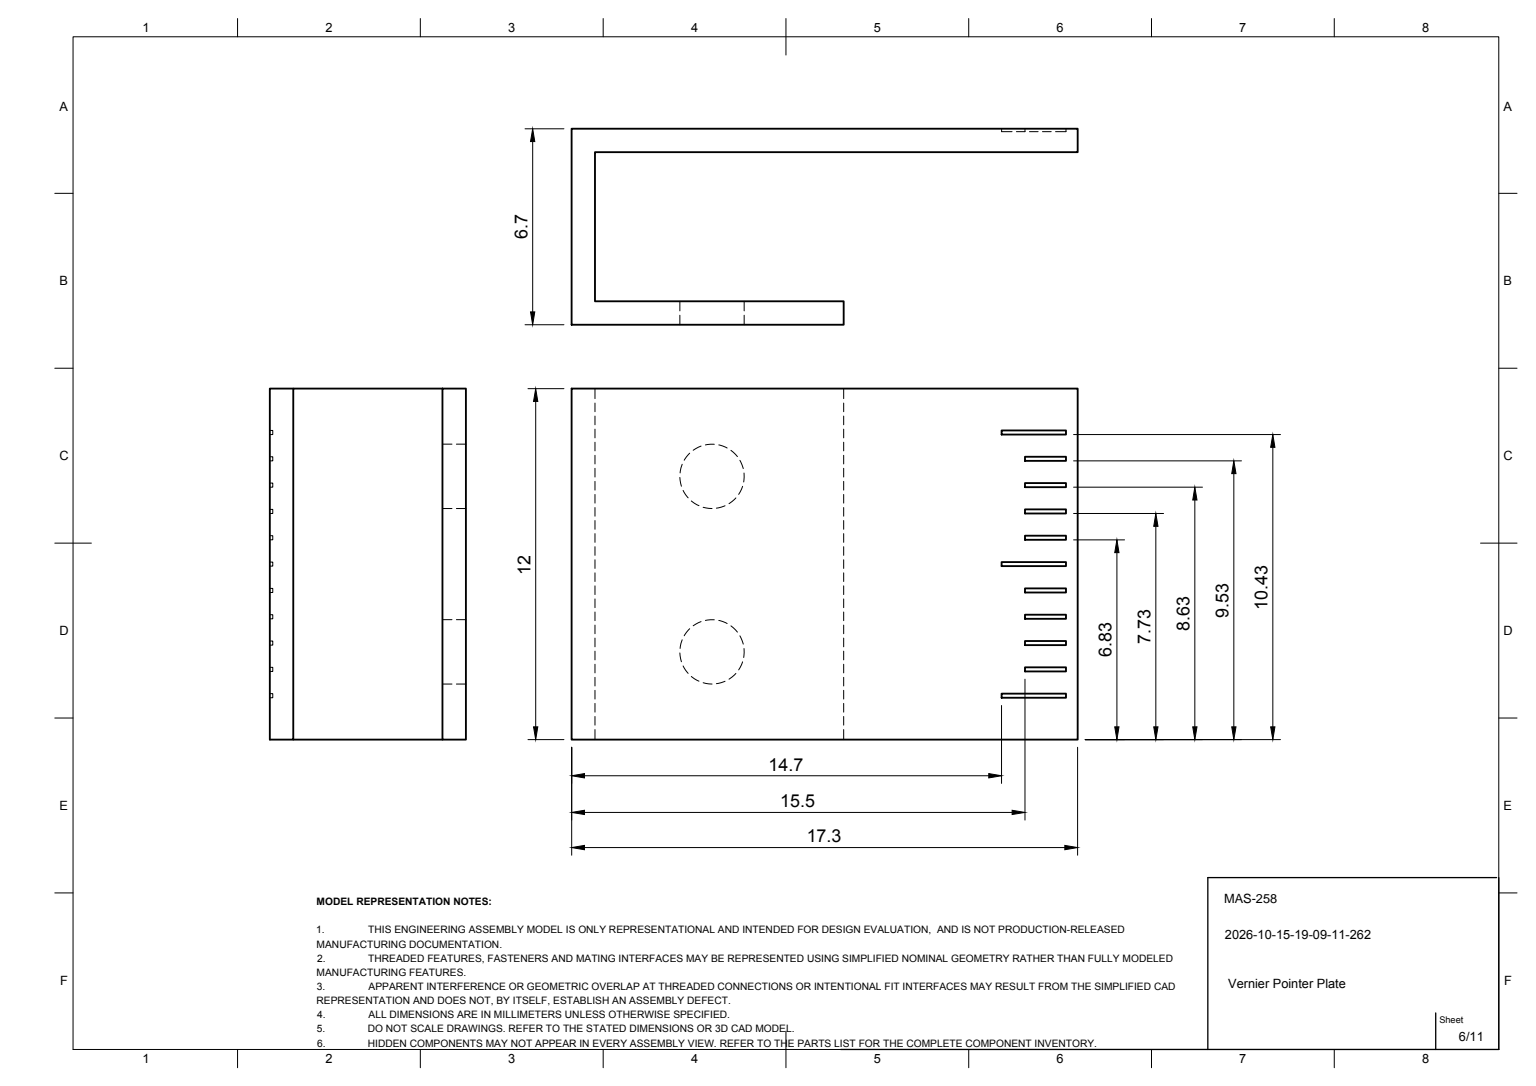
ISO-10303-21;
HEADER;
/* Generated by software containing ST-Developer
 * from STEP Tools, Inc. (www.steptools.com) 
 */

FILE_DESCRIPTION(
/* description */ (''),
/* implementation_level */ '2;1');

FILE_NAME(
/* name */ 'Vernier Pointer Plate.step',
/* time_stamp */ '2026-10-15T12:29:06-07:00',
/* author */ (''),
/* organization */ (''),
/* preprocessor_version */ 'ST-DEVELOPER v20.2',
/* originating_system */ 'Autodesk Translation Framework v15.15.0.0',
/* authorisation */ '');

FILE_SCHEMA (('AUTOMOTIVE_DESIGN { 1 0 10303 214 3 1 1 }'));
ENDSEC;

DATA;
#10=MECHANICAL_DESIGN_GEOMETRIC_PRESENTATION_REPRESENTATION('',(#1745),#135282);
#1719=SHAPE_REPRESENTATION_RELATIONSHIP('SRR','None',#135343,#1732);
#1732=ADVANCED_BREP_SHAPE_REPRESENTATION('',(#1758),#135275);
#1745=STYLED_ITEM('',(#135417),#1758);
#1758=MANIFOLD_SOLID_BREP('Body1',#32081);
#1846=CYLINDRICAL_SURFACE('',#33343,1.1);
#1847=CYLINDRICAL_SURFACE('',#33346,1.1);
#2195=FACE_BOUND('',#6494,.T.);
#2196=FACE_BOUND('',#6495,.T.);
#2197=FACE_BOUND('',#6498,.T.);
#2198=FACE_BOUND('',#6499,.T.);
#2199=FACE_BOUND('',#6504,.T.);
#2200=FACE_BOUND('',#6505,.T.);
#2201=FACE_BOUND('',#6506,.T.);
#2202=FACE_BOUND('',#6507,.T.);
#2203=FACE_BOUND('',#6508,.T.);
#2204=FACE_BOUND('',#6509,.T.);
#2205=FACE_BOUND('',#6510,.T.);
#2206=FACE_BOUND('',#6511,.T.);
#2207=FACE_BOUND('',#6512,.T.);
#2208=FACE_BOUND('',#6513,.T.);
#2209=FACE_BOUND('',#6514,.T.);
#2961=PLANE('',#33288);
#2962=PLANE('',#33289);
#2963=PLANE('',#33290);
#2964=PLANE('',#33291);
#2965=PLANE('',#33292);
#2966=PLANE('',#33293);
#2967=PLANE('',#33294);
#2968=PLANE('',#33295);
#2969=PLANE('',#33296);
#2970=PLANE('',#33297);
#2971=PLANE('',#33298);
#2972=PLANE('',#33299);
#2973=PLANE('',#33300);
#2974=PLANE('',#33301);
#2975=PLANE('',#33302);
#2976=PLANE('',#33303);
#2977=PLANE('',#33304);
#2978=PLANE('',#33305);
#2979=PLANE('',#33306);
#2980=PLANE('',#33307);
#2981=PLANE('',#33308);
#2982=PLANE('',#33309);
#2983=PLANE('',#33310);
#2984=PLANE('',#33311);
#2985=PLANE('',#33312);
#2986=PLANE('',#33313);
#2987=PLANE('',#33314);
#2988=PLANE('',#33315);
#2989=PLANE('',#33316);
#2990=PLANE('',#33317);
#2991=PLANE('',#33318);
#2992=PLANE('',#33319);
#2993=PLANE('',#33320);
#2994=PLANE('',#33321);
#2995=PLANE('',#33322);
#2996=PLANE('',#33323);
#2997=PLANE('',#33324);
#2998=PLANE('',#33325);
#2999=PLANE('',#33326);
#3000=PLANE('',#33327);
#3001=PLANE('',#33328);
#3002=PLANE('',#33329);
#3003=PLANE('',#33330);
#3004=PLANE('',#33331);
#3005=PLANE('',#33332);
#3006=PLANE('',#33333);
#3007=PLANE('',#33334);
#3008=PLANE('',#33335);
#3009=PLANE('',#33336);
#3010=PLANE('',#33337);
#3011=PLANE('',#33338);
#3012=PLANE('',#33339);
#3013=PLANE('',#33340);
#3014=PLANE('',#33341);
#3015=PLANE('',#33342);
#3016=PLANE('',#33349);
#3017=PLANE('',#33350);
#3018=PLANE('',#33351);
#3019=PLANE('',#33352);
#3020=PLANE('',#33353);
#3021=PLANE('',#33354);
#3022=PLANE('',#33355);
#3023=PLANE('',#33356);
#3024=PLANE('',#33357);
#3025=PLANE('',#33358);
#4503=FACE_OUTER_BOUND('',#6436,.T.);
#4504=FACE_OUTER_BOUND('',#6437,.T.);
#4505=FACE_OUTER_BOUND('',#6438,.T.);
#4506=FACE_OUTER_BOUND('',#6439,.T.);
#4507=FACE_OUTER_BOUND('',#6440,.T.);
#4508=FACE_OUTER_BOUND('',#6441,.T.);
#4509=FACE_OUTER_BOUND('',#6442,.T.);
#4510=FACE_OUTER_BOUND('',#6443,.T.);
#4511=FACE_OUTER_BOUND('',#6444,.T.);
#4512=FACE_OUTER_BOUND('',#6445,.T.);
#4513=FACE_OUTER_BOUND('',#6446,.T.);
#4514=FACE_OUTER_BOUND('',#6447,.T.);
#4515=FACE_OUTER_BOUND('',#6448,.T.);
#4516=FACE_OUTER_BOUND('',#6449,.T.);
#4517=FACE_OUTER_BOUND('',#6450,.T.);
#4518=FACE_OUTER_BOUND('',#6451,.T.);
#4519=FACE_OUTER_BOUND('',#6452,.T.);
#4520=FACE_OUTER_BOUND('',#6453,.T.);
#4521=FACE_OUTER_BOUND('',#6454,.T.);
#4522=FACE_OUTER_BOUND('',#6455,.T.);
#4523=FACE_OUTER_BOUND('',#6456,.T.);
#4524=FACE_OUTER_BOUND('',#6457,.T.);
#4525=FACE_OUTER_BOUND('',#6458,.T.);
#4526=FACE_OUTER_BOUND('',#6459,.T.);
#4527=FACE_OUTER_BOUND('',#6460,.T.);
#4528=FACE_OUTER_BOUND('',#6461,.T.);
#4529=FACE_OUTER_BOUND('',#6462,.T.);
#4530=FACE_OUTER_BOUND('',#6463,.T.);
#4531=FACE_OUTER_BOUND('',#6464,.T.);
#4532=FACE_OUTER_BOUND('',#6465,.T.);
#4533=FACE_OUTER_BOUND('',#6466,.T.);
#4534=FACE_OUTER_BOUND('',#6467,.T.);
#4535=FACE_OUTER_BOUND('',#6468,.T.);
#4536=FACE_OUTER_BOUND('',#6469,.T.);
#4537=FACE_OUTER_BOUND('',#6470,.T.);
#4538=FACE_OUTER_BOUND('',#6471,.T.);
#4539=FACE_OUTER_BOUND('',#6472,.T.);
#4540=FACE_OUTER_BOUND('',#6473,.T.);
#4541=FACE_OUTER_BOUND('',#6474,.T.);
#4542=FACE_OUTER_BOUND('',#6475,.T.);
#4543=FACE_OUTER_BOUND('',#6476,.T.);
#4544=FACE_OUTER_BOUND('',#6477,.T.);
#4545=FACE_OUTER_BOUND('',#6478,.T.);
#4546=FACE_OUTER_BOUND('',#6479,.T.);
#4547=FACE_OUTER_BOUND('',#6480,.T.);
#4548=FACE_OUTER_BOUND('',#6481,.T.);
#4549=FACE_OUTER_BOUND('',#6482,.T.);
#4550=FACE_OUTER_BOUND('',#6483,.T.);
#4551=FACE_OUTER_BOUND('',#6484,.T.);
#4552=FACE_OUTER_BOUND('',#6485,.T.);
#4553=FACE_OUTER_BOUND('',#6486,.T.);
#4554=FACE_OUTER_BOUND('',#6487,.T.);
#4555=FACE_OUTER_BOUND('',#6488,.T.);
#4556=FACE_OUTER_BOUND('',#6489,.T.);
#4557=FACE_OUTER_BOUND('',#6490,.T.);
#4558=FACE_OUTER_BOUND('',#6491,.T.);
#4559=FACE_OUTER_BOUND('',#6492,.T.);
#4560=FACE_OUTER_BOUND('',#6493,.T.);
#4561=FACE_OUTER_BOUND('',#6496,.T.);
#4562=FACE_OUTER_BOUND('',#6497,.T.);
#4563=FACE_OUTER_BOUND('',#6500,.T.);
#4564=FACE_OUTER_BOUND('',#6501,.T.);
#4565=FACE_OUTER_BOUND('',#6502,.T.);
#4566=FACE_OUTER_BOUND('',#6503,.T.);
#4567=FACE_OUTER_BOUND('',#6515,.T.);
#4568=FACE_OUTER_BOUND('',#6516,.T.);
#4569=FACE_OUTER_BOUND('',#6517,.T.);
#6436=EDGE_LOOP('',(#26862,#26863,#26864,#26865));
#6437=EDGE_LOOP('',(#26866,#26867,#26868,#26869));
#6438=EDGE_LOOP('',(#26870,#26871,#26872,#26873));
#6439=EDGE_LOOP('',(#26874,#26875,#26876,#26877));
#6440=EDGE_LOOP('',(#26878,#26879,#26880,#26881));
#6441=EDGE_LOOP('',(#26882,#26883,#26884,#26885));
#6442=EDGE_LOOP('',(#26886,#26887,#26888,#26889));
#6443=EDGE_LOOP('',(#26890,#26891,#26892,#26893));
#6444=EDGE_LOOP('',(#26894,#26895,#26896,#26897));
#6445=EDGE_LOOP('',(#26898,#26899,#26900,#26901));
#6446=EDGE_LOOP('',(#26902,#26903,#26904,#26905));
#6447=EDGE_LOOP('',(#26906,#26907,#26908,#26909));
#6448=EDGE_LOOP('',(#26910,#26911,#26912,#26913));
#6449=EDGE_LOOP('',(#26914,#26915,#26916,#26917));
#6450=EDGE_LOOP('',(#26918,#26919,#26920,#26921));
#6451=EDGE_LOOP('',(#26922,#26923,#26924,#26925));
#6452=EDGE_LOOP('',(#26926,#26927,#26928,#26929));
#6453=EDGE_LOOP('',(#26930,#26931,#26932,#26933));
#6454=EDGE_LOOP('',(#26934,#26935,#26936,#26937));
#6455=EDGE_LOOP('',(#26938,#26939,#26940,#26941));
#6456=EDGE_LOOP('',(#26942,#26943,#26944,#26945));
#6457=EDGE_LOOP('',(#26946,#26947,#26948,#26949));
#6458=EDGE_LOOP('',(#26950,#26951,#26952,#26953));
#6459=EDGE_LOOP('',(#26954,#26955,#26956,#26957));
#6460=EDGE_LOOP('',(#26958,#26959,#26960,#26961));
#6461=EDGE_LOOP('',(#26962,#26963,#26964,#26965));
#6462=EDGE_LOOP('',(#26966,#26967,#26968,#26969));
#6463=EDGE_LOOP('',(#26970,#26971,#26972,#26973));
#6464=EDGE_LOOP('',(#26974,#26975,#26976,#26977));
#6465=EDGE_LOOP('',(#26978,#26979,#26980,#26981));
#6466=EDGE_LOOP('',(#26982,#26983,#26984,#26985));
#6467=EDGE_LOOP('',(#26986,#26987,#26988,#26989));
#6468=EDGE_LOOP('',(#26990,#26991,#26992,#26993));
#6469=EDGE_LOOP('',(#26994,#26995,#26996,#26997));
#6470=EDGE_LOOP('',(#26998,#26999,#27000,#27001));
#6471=EDGE_LOOP('',(#27002,#27003,#27004,#27005));
#6472=EDGE_LOOP('',(#27006,#27007,#27008,#27009));
#6473=EDGE_LOOP('',(#27010,#27011,#27012,#27013));
#6474=EDGE_LOOP('',(#27014,#27015,#27016,#27017));
#6475=EDGE_LOOP('',(#27018,#27019,#27020,#27021));
#6476=EDGE_LOOP('',(#27022,#27023,#27024,#27025));
#6477=EDGE_LOOP('',(#27026,#27027,#27028,#27029));
#6478=EDGE_LOOP('',(#27030,#27031,#27032,#27033));
#6479=EDGE_LOOP('',(#27034,#27035,#27036,#27037));
#6480=EDGE_LOOP('',(#27038,#27039,#27040,#27041));
#6481=EDGE_LOOP('',(#27042,#27043,#27044,#27045));
#6482=EDGE_LOOP('',(#27046,#27047,#27048,#27049));
#6483=EDGE_LOOP('',(#27050,#27051,#27052,#27053));
#6484=EDGE_LOOP('',(#27054,#27055,#27056,#27057));
#6485=EDGE_LOOP('',(#27058,#27059,#27060,#27061));
#6486=EDGE_LOOP('',(#27062,#27063,#27064,#27065));
#6487=EDGE_LOOP('',(#27066,#27067,#27068,#27069));
#6488=EDGE_LOOP('',(#27070,#27071,#27072,#27073));
#6489=EDGE_LOOP('',(#27074,#27075,#27076,#27077));
#6490=EDGE_LOOP('',(#27078,#27079,#27080,#27081));
#6491=EDGE_LOOP('',(#27082,#27083,#27084,#27085));
#6492=EDGE_LOOP('',(#27086,#27087,#27088,#27089));
#6493=EDGE_LOOP('',(#27090,#27091,#27092,#27093));
#6494=EDGE_LOOP('',(#27094));
#6495=EDGE_LOOP('',(#27095));
#6496=EDGE_LOOP('',(#27096,#27097,#27098,#27099));
#6497=EDGE_LOOP('',(#27100,#27101,#27102,#27103));
#6498=EDGE_LOOP('',(#27104));
#6499=EDGE_LOOP('',(#27105));
#6500=EDGE_LOOP('',(#27106,#27107,#27108,#27109));
#6501=EDGE_LOOP('',(#27110,#27111,#27112,#27113));
#6502=EDGE_LOOP('',(#27114,#27115,#27116,#27117));
#6503=EDGE_LOOP('',(#27118,#27119,#27120,#27121));
#6504=EDGE_LOOP('',(#27122,#27123,#27124,#27125));
#6505=EDGE_LOOP('',(#27126,#27127,#27128,#27129));
#6506=EDGE_LOOP('',(#27130,#27131,#27132,#27133));
#6507=EDGE_LOOP('',(#27134,#27135,#27136,#27137));
#6508=EDGE_LOOP('',(#27138,#27139,#27140,#27141));
#6509=EDGE_LOOP('',(#27142,#27143,#27144,#27145));
#6510=EDGE_LOOP('',(#27146,#27147,#27148,#27149));
#6511=EDGE_LOOP('',(#27150,#27151,#27152,#27153));
#6512=EDGE_LOOP('',(#27154,#27155,#27156,#27157));
#6513=EDGE_LOOP('',(#27158,#27159,#27160,#27161));
#6514=EDGE_LOOP('',(#27162,#27163,#27164,#27165));
#6515=EDGE_LOOP('',(#27166,#27167,#27168,#27169));
#6516=EDGE_LOOP('',(#27170,#27171,#27172,#27173,#27174,#27175,#27176,#27177));
#6517=EDGE_LOOP('',(#27178,#27179,#27180,#27181,#27182,#27183,#27184,#27185));
#9058=LINE('',#76652,#11895);
#9059=LINE('',#76654,#11896);
#9060=LINE('',#76656,#11897);
#9061=LINE('',#76657,#11898);
#9062=LINE('',#76660,#11899);
#9063=LINE('',#76662,#11900);
#9064=LINE('',#76663,#11901);
#9065=LINE('',#76666,#11902);
#9066=LINE('',#76668,#11903);
#9067=LINE('',#76669,#11904);
#9068=LINE('',#76671,#11905);
#9069=LINE('',#76672,#11906);
#9070=LINE('',#76677,#11907);
#9071=LINE('',#76679,#11908);
#9072=LINE('',#76681,#11909);
#9073=LINE('',#76682,#11910);
#9074=LINE('',#76685,#11911);
#9075=LINE('',#76687,#11912);
#9076=LINE('',#76688,#11913);
#9077=LINE('',#76691,#11914);
#9078=LINE('',#76693,#11915);
#9079=LINE('',#76694,#11916);
#9080=LINE('',#76696,#11917);
#9081=LINE('',#76697,#11918);
#9082=LINE('',#76702,#11919);
#9083=LINE('',#76704,#11920);
#9084=LINE('',#76706,#11921);
#9085=LINE('',#76707,#11922);
#9086=LINE('',#76710,#11923);
#9087=LINE('',#76712,#11924);
#9088=LINE('',#76713,#11925);
#9089=LINE('',#76716,#11926);
#9090=LINE('',#76718,#11927);
#9091=LINE('',#76719,#11928);
#9092=LINE('',#76721,#11929);
#9093=LINE('',#76722,#11930);
#9094=LINE('',#76727,#11931);
#9095=LINE('',#76729,#11932);
#9096=LINE('',#76731,#11933);
#9097=LINE('',#76732,#11934);
#9098=LINE('',#76735,#11935);
#9099=LINE('',#76737,#11936);
#9100=LINE('',#76738,#11937);
#9101=LINE('',#76741,#11938);
#9102=LINE('',#76743,#11939);
#9103=LINE('',#76744,#11940);
#9104=LINE('',#76746,#11941);
#9105=LINE('',#76747,#11942);
#9106=LINE('',#76752,#11943);
#9107=LINE('',#76754,#11944);
#9108=LINE('',#76756,#11945);
#9109=LINE('',#76757,#11946);
#9110=LINE('',#76760,#11947);
#9111=LINE('',#76762,#11948);
#9112=LINE('',#76763,#11949);
#9113=LINE('',#76766,#11950);
#9114=LINE('',#76768,#11951);
#9115=LINE('',#76769,#11952);
#9116=LINE('',#76771,#11953);
#9117=LINE('',#76772,#11954);
#9118=LINE('',#76777,#11955);
#9119=LINE('',#76779,#11956);
#9120=LINE('',#76781,#11957);
#9121=LINE('',#76782,#11958);
#9122=LINE('',#76785,#11959);
#9123=LINE('',#76787,#11960);
#9124=LINE('',#76788,#11961);
#9125=LINE('',#76791,#11962);
#9126=LINE('',#76793,#11963);
#9127=LINE('',#76794,#11964);
#9128=LINE('',#76796,#11965);
#9129=LINE('',#76797,#11966);
#9130=LINE('',#76802,#11967);
#9131=LINE('',#76804,#11968);
#9132=LINE('',#76806,#11969);
#9133=LINE('',#76807,#11970);
#9134=LINE('',#76810,#11971);
#9135=LINE('',#76812,#11972);
#9136=LINE('',#76813,#11973);
#9137=LINE('',#76816,#11974);
#9138=LINE('',#76818,#11975);
#9139=LINE('',#76819,#11976);
#9140=LINE('',#76821,#11977);
#9141=LINE('',#76822,#11978);
#9142=LINE('',#76827,#11979);
#9143=LINE('',#76829,#11980);
#9144=LINE('',#76831,#11981);
#9145=LINE('',#76832,#11982);
#9146=LINE('',#76835,#11983);
#9147=LINE('',#76837,#11984);
#9148=LINE('',#76838,#11985);
#9149=LINE('',#76841,#11986);
#9150=LINE('',#76843,#11987);
#9151=LINE('',#76844,#11988);
#9152=LINE('',#76846,#11989);
#9153=LINE('',#76847,#11990);
#9154=LINE('',#76852,#11991);
#9155=LINE('',#76854,#11992);
#9156=LINE('',#76856,#11993);
#9157=LINE('',#76857,#11994);
#9158=LINE('',#76860,#11995);
#9159=LINE('',#76862,#11996);
#9160=LINE('',#76863,#11997);
#9161=LINE('',#76866,#11998);
#9162=LINE('',#76868,#11999);
#9163=LINE('',#76869,#12000);
#9164=LINE('',#76871,#12001);
#9165=LINE('',#76872,#12002);
#9166=LINE('',#76877,#12003);
#9167=LINE('',#76879,#12004);
#9168=LINE('',#76881,#12005);
#9169=LINE('',#76882,#12006);
#9170=LINE('',#76885,#12007);
#9171=LINE('',#76887,#12008);
#9172=LINE('',#76888,#12009);
#9173=LINE('',#76891,#12010);
#9174=LINE('',#76893,#12011);
#9175=LINE('',#76894,#12012);
#9176=LINE('',#76896,#12013);
#9177=LINE('',#76897,#12014);
#9178=LINE('',#76902,#12015);
#9179=LINE('',#76904,#12016);
#9180=LINE('',#76906,#12017);
#9181=LINE('',#76907,#12018);
#9182=LINE('',#76910,#12019);
#9183=LINE('',#76912,#12020);
#9184=LINE('',#76913,#12021);
#9185=LINE('',#76916,#12022);
#9186=LINE('',#76918,#12023);
#9187=LINE('',#76919,#12024);
#9188=LINE('',#76921,#12025);
#9189=LINE('',#76922,#12026);
#9190=LINE('',#76928,#12027);
#9191=LINE('',#76934,#12028);
#9192=LINE('',#76939,#12029);
#9193=LINE('',#76941,#12030);
#9194=LINE('',#76943,#12031);
#9195=LINE('',#76944,#12032);
#9196=LINE('',#76947,#12033);
#9197=LINE('',#76949,#12034);
#9198=LINE('',#76950,#12035);
#9199=LINE('',#76953,#12036);
#9200=LINE('',#76955,#12037);
#9201=LINE('',#76956,#12038);
#9202=LINE('',#76959,#12039);
#9203=LINE('',#76961,#12040);
#9204=LINE('',#76962,#12041);
#9205=LINE('',#76965,#12042);
#9206=LINE('',#76967,#12043);
#9207=LINE('',#76968,#12044);
#9208=LINE('',#76971,#12045);
#9209=LINE('',#76973,#12046);
#9210=LINE('',#76974,#12047);
#9211=LINE('',#76977,#12048);
#9212=LINE('',#76979,#12049);
#9213=LINE('',#76980,#12050);
#9214=LINE('',#76982,#12051);
#9215=LINE('',#76983,#12052);
#11895=VECTOR('',#38326,10.);
#11896=VECTOR('',#38327,10.);
#11897=VECTOR('',#38328,10.);
#11898=VECTOR('',#38329,10.);
#11899=VECTOR('',#38332,10.);
#11900=VECTOR('',#38333,10.);
#11901=VECTOR('',#38334,10.);
#11902=VECTOR('',#38337,10.);
#11903=VECTOR('',#38338,10.);
#11904=VECTOR('',#38339,10.);
#11905=VECTOR('',#38342,10.);
#11906=VECTOR('',#38343,10.);
#11907=VECTOR('',#38348,10.);
#11908=VECTOR('',#38349,10.);
#11909=VECTOR('',#38350,10.);
#11910=VECTOR('',#38351,10.);
#11911=VECTOR('',#38354,10.);
#11912=VECTOR('',#38355,10.);
#11913=VECTOR('',#38356,10.);
#11914=VECTOR('',#38359,10.);
#11915=VECTOR('',#38360,10.);
#11916=VECTOR('',#38361,10.);
#11917=VECTOR('',#38364,10.);
#11918=VECTOR('',#38365,10.);
#11919=VECTOR('',#38370,10.);
#11920=VECTOR('',#38371,10.);
#11921=VECTOR('',#38372,10.);
#11922=VECTOR('',#38373,10.);
#11923=VECTOR('',#38376,10.);
#11924=VECTOR('',#38377,10.);
#11925=VECTOR('',#38378,10.);
#11926=VECTOR('',#38381,10.);
#11927=VECTOR('',#38382,10.);
#11928=VECTOR('',#38383,10.);
#11929=VECTOR('',#38386,10.);
#11930=VECTOR('',#38387,10.);
#11931=VECTOR('',#38392,10.);
#11932=VECTOR('',#38393,10.);
#11933=VECTOR('',#38394,10.);
#11934=VECTOR('',#38395,10.);
#11935=VECTOR('',#38398,10.);
#11936=VECTOR('',#38399,10.);
#11937=VECTOR('',#38400,10.);
#11938=VECTOR('',#38403,10.);
#11939=VECTOR('',#38404,10.);
#11940=VECTOR('',#38405,10.);
#11941=VECTOR('',#38408,10.);
#11942=VECTOR('',#38409,10.);
#11943=VECTOR('',#38414,10.);
#11944=VECTOR('',#38415,10.);
#11945=VECTOR('',#38416,10.);
#11946=VECTOR('',#38417,10.);
#11947=VECTOR('',#38420,10.);
#11948=VECTOR('',#38421,10.);
#11949=VECTOR('',#38422,10.);
#11950=VECTOR('',#38425,10.);
#11951=VECTOR('',#38426,10.);
#11952=VECTOR('',#38427,10.);
#11953=VECTOR('',#38430,10.);
#11954=VECTOR('',#38431,10.);
#11955=VECTOR('',#38436,10.);
#11956=VECTOR('',#38437,10.);
#11957=VECTOR('',#38438,10.);
#11958=VECTOR('',#38439,10.);
#11959=VECTOR('',#38442,10.);
#11960=VECTOR('',#38443,10.);
#11961=VECTOR('',#38444,10.);
#11962=VECTOR('',#38447,10.);
#11963=VECTOR('',#38448,10.);
#11964=VECTOR('',#38449,10.);
#11965=VECTOR('',#38452,10.);
#11966=VECTOR('',#38453,10.);
#11967=VECTOR('',#38458,10.);
#11968=VECTOR('',#38459,10.);
#11969=VECTOR('',#38460,10.);
#11970=VECTOR('',#38461,10.);
#11971=VECTOR('',#38464,10.);
#11972=VECTOR('',#38465,10.);
#11973=VECTOR('',#38466,10.);
#11974=VECTOR('',#38469,10.);
#11975=VECTOR('',#38470,10.);
#11976=VECTOR('',#38471,10.);
#11977=VECTOR('',#38474,10.);
#11978=VECTOR('',#38475,10.);
#11979=VECTOR('',#38480,10.);
#11980=VECTOR('',#38481,10.);
#11981=VECTOR('',#38482,10.);
#11982=VECTOR('',#38483,10.);
#11983=VECTOR('',#38486,10.);
#11984=VECTOR('',#38487,10.);
#11985=VECTOR('',#38488,10.);
#11986=VECTOR('',#38491,10.);
#11987=VECTOR('',#38492,10.);
#11988=VECTOR('',#38493,10.);
#11989=VECTOR('',#38496,10.);
#11990=VECTOR('',#38497,10.);
#11991=VECTOR('',#38502,10.);
#11992=VECTOR('',#38503,10.);
#11993=VECTOR('',#38504,10.);
#11994=VECTOR('',#38505,10.);
#11995=VECTOR('',#38508,10.);
#11996=VECTOR('',#38509,10.);
#11997=VECTOR('',#38510,10.);
#11998=VECTOR('',#38513,10.);
#11999=VECTOR('',#38514,10.);
#12000=VECTOR('',#38515,10.);
#12001=VECTOR('',#38518,10.);
#12002=VECTOR('',#38519,10.);
#12003=VECTOR('',#38524,10.);
#12004=VECTOR('',#38525,10.);
#12005=VECTOR('',#38526,10.);
#12006=VECTOR('',#38527,10.);
#12007=VECTOR('',#38530,10.);
#12008=VECTOR('',#38531,10.);
#12009=VECTOR('',#38532,10.);
#12010=VECTOR('',#38535,10.);
#12011=VECTOR('',#38536,10.);
#12012=VECTOR('',#38537,10.);
#12013=VECTOR('',#38540,10.);
#12014=VECTOR('',#38541,10.);
#12015=VECTOR('',#38546,10.);
#12016=VECTOR('',#38547,10.);
#12017=VECTOR('',#38548,10.);
#12018=VECTOR('',#38549,10.);
#12019=VECTOR('',#38552,10.);
#12020=VECTOR('',#38553,10.);
#12021=VECTOR('',#38554,10.);
#12022=VECTOR('',#38557,10.);
#12023=VECTOR('',#38558,10.);
#12024=VECTOR('',#38559,10.);
#12025=VECTOR('',#38562,10.);
#12026=VECTOR('',#38563,10.);
#12027=VECTOR('',#38570,1.1);
#12028=VECTOR('',#38577,1.1);
#12029=VECTOR('',#38582,10.);
#12030=VECTOR('',#38583,10.);
#12031=VECTOR('',#38584,10.);
#12032=VECTOR('',#38585,10.);
#12033=VECTOR('',#38588,10.);
#12034=VECTOR('',#38589,10.);
#12035=VECTOR('',#38590,10.);
#12036=VECTOR('',#38593,10.);
#12037=VECTOR('',#38594,10.);
#12038=VECTOR('',#38595,10.);
#12039=VECTOR('',#38598,10.);
#12040=VECTOR('',#38599,10.);
#12041=VECTOR('',#38600,10.);
#12042=VECTOR('',#38603,10.);
#12043=VECTOR('',#38604,10.);
#12044=VECTOR('',#38605,10.);
#12045=VECTOR('',#38608,10.);
#12046=VECTOR('',#38609,10.);
#12047=VECTOR('',#38610,10.);
#12048=VECTOR('',#38613,10.);
#12049=VECTOR('',#38614,10.);
#12050=VECTOR('',#38615,10.);
#12051=VECTOR('',#38618,10.);
#12052=VECTOR('',#38619,10.);
#12928=CIRCLE('',#33344,1.1);
#12929=CIRCLE('',#33345,1.1);
#12930=CIRCLE('',#33347,1.1);
#12931=CIRCLE('',#33348,1.1);
#15209=VERTEX_POINT('',#76650);
#15210=VERTEX_POINT('',#76651);
#15211=VERTEX_POINT('',#76653);
#15212=VERTEX_POINT('',#76655);
#15213=VERTEX_POINT('',#76659);
#15214=VERTEX_POINT('',#76661);
#15215=VERTEX_POINT('',#76665);
#15216=VERTEX_POINT('',#76667);
#15217=VERTEX_POINT('',#76675);
#15218=VERTEX_POINT('',#76676);
#15219=VERTEX_POINT('',#76678);
#15220=VERTEX_POINT('',#76680);
#15221=VERTEX_POINT('',#76684);
#15222=VERTEX_POINT('',#76686);
#15223=VERTEX_POINT('',#76690);
#15224=VERTEX_POINT('',#76692);
#15225=VERTEX_POINT('',#76700);
#15226=VERTEX_POINT('',#76701);
#15227=VERTEX_POINT('',#76703);
#15228=VERTEX_POINT('',#76705);
#15229=VERTEX_POINT('',#76709);
#15230=VERTEX_POINT('',#76711);
#15231=VERTEX_POINT('',#76715);
#15232=VERTEX_POINT('',#76717);
#15233=VERTEX_POINT('',#76725);
#15234=VERTEX_POINT('',#76726);
#15235=VERTEX_POINT('',#76728);
#15236=VERTEX_POINT('',#76730);
#15237=VERTEX_POINT('',#76734);
#15238=VERTEX_POINT('',#76736);
#15239=VERTEX_POINT('',#76740);
#15240=VERTEX_POINT('',#76742);
#15241=VERTEX_POINT('',#76750);
#15242=VERTEX_POINT('',#76751);
#15243=VERTEX_POINT('',#76753);
#15244=VERTEX_POINT('',#76755);
#15245=VERTEX_POINT('',#76759);
#15246=VERTEX_POINT('',#76761);
#15247=VERTEX_POINT('',#76765);
#15248=VERTEX_POINT('',#76767);
#15249=VERTEX_POINT('',#76775);
#15250=VERTEX_POINT('',#76776);
#15251=VERTEX_POINT('',#76778);
#15252=VERTEX_POINT('',#76780);
#15253=VERTEX_POINT('',#76784);
#15254=VERTEX_POINT('',#76786);
#15255=VERTEX_POINT('',#76790);
#15256=VERTEX_POINT('',#76792);
#15257=VERTEX_POINT('',#76800);
#15258=VERTEX_POINT('',#76801);
#15259=VERTEX_POINT('',#76803);
#15260=VERTEX_POINT('',#76805);
#15261=VERTEX_POINT('',#76809);
#15262=VERTEX_POINT('',#76811);
#15263=VERTEX_POINT('',#76815);
#15264=VERTEX_POINT('',#76817);
#15265=VERTEX_POINT('',#76825);
#15266=VERTEX_POINT('',#76826);
#15267=VERTEX_POINT('',#76828);
#15268=VERTEX_POINT('',#76830);
#15269=VERTEX_POINT('',#76834);
#15270=VERTEX_POINT('',#76836);
#15271=VERTEX_POINT('',#76840);
#15272=VERTEX_POINT('',#76842);
#15273=VERTEX_POINT('',#76850);
#15274=VERTEX_POINT('',#76851);
#15275=VERTEX_POINT('',#76853);
#15276=VERTEX_POINT('',#76855);
#15277=VERTEX_POINT('',#76859);
#15278=VERTEX_POINT('',#76861);
#15279=VERTEX_POINT('',#76865);
#15280=VERTEX_POINT('',#76867);
#15281=VERTEX_POINT('',#76875);
#15282=VERTEX_POINT('',#76876);
#15283=VERTEX_POINT('',#76878);
#15284=VERTEX_POINT('',#76880);
#15285=VERTEX_POINT('',#76884);
#15286=VERTEX_POINT('',#76886);
#15287=VERTEX_POINT('',#76890);
#15288=VERTEX_POINT('',#76892);
#15289=VERTEX_POINT('',#76900);
#15290=VERTEX_POINT('',#76901);
#15291=VERTEX_POINT('',#76903);
#15292=VERTEX_POINT('',#76905);
#15293=VERTEX_POINT('',#76909);
#15294=VERTEX_POINT('',#76911);
#15295=VERTEX_POINT('',#76915);
#15296=VERTEX_POINT('',#76917);
#15297=VERTEX_POINT('',#76925);
#15298=VERTEX_POINT('',#76927);
#15299=VERTEX_POINT('',#76931);
#15300=VERTEX_POINT('',#76933);
#15301=VERTEX_POINT('',#76937);
#15302=VERTEX_POINT('',#76938);
#15303=VERTEX_POINT('',#76940);
#15304=VERTEX_POINT('',#76942);
#15305=VERTEX_POINT('',#76946);
#15306=VERTEX_POINT('',#76948);
#15307=VERTEX_POINT('',#76952);
#15308=VERTEX_POINT('',#76954);
#15309=VERTEX_POINT('',#76958);
#15310=VERTEX_POINT('',#76960);
#15311=VERTEX_POINT('',#76964);
#15312=VERTEX_POINT('',#76966);
#15313=VERTEX_POINT('',#76970);
#15314=VERTEX_POINT('',#76972);
#15315=VERTEX_POINT('',#76976);
#15316=VERTEX_POINT('',#76978);
#19282=EDGE_CURVE('',#15209,#15210,#9058,.T.);
#19283=EDGE_CURVE('',#15209,#15211,#9059,.T.);
#19284=EDGE_CURVE('',#15211,#15212,#9060,.T.);
#19285=EDGE_CURVE('',#15210,#15212,#9061,.T.);
#19286=EDGE_CURVE('',#15213,#15209,#9062,.T.);
#19287=EDGE_CURVE('',#15213,#15214,#9063,.T.);
#19288=EDGE_CURVE('',#15214,#15211,#9064,.T.);
#19289=EDGE_CURVE('',#15215,#15213,#9065,.T.);
#19290=EDGE_CURVE('',#15215,#15216,#9066,.T.);
#19291=EDGE_CURVE('',#15216,#15214,#9067,.T.);
#19292=EDGE_CURVE('',#15210,#15215,#9068,.T.);
#19293=EDGE_CURVE('',#15212,#15216,#9069,.T.);
#19294=EDGE_CURVE('',#15217,#15218,#9070,.T.);
#19295=EDGE_CURVE('',#15217,#15219,#9071,.T.);
#19296=EDGE_CURVE('',#15219,#15220,#9072,.T.);
#19297=EDGE_CURVE('',#15218,#15220,#9073,.T.);
#19298=EDGE_CURVE('',#15221,#15217,#9074,.T.);
#19299=EDGE_CURVE('',#15221,#15222,#9075,.T.);
#19300=EDGE_CURVE('',#15222,#15219,#9076,.T.);
#19301=EDGE_CURVE('',#15223,#15221,#9077,.T.);
#19302=EDGE_CURVE('',#15223,#15224,#9078,.T.);
#19303=EDGE_CURVE('',#15224,#15222,#9079,.T.);
#19304=EDGE_CURVE('',#15218,#15223,#9080,.T.);
#19305=EDGE_CURVE('',#15220,#15224,#9081,.T.);
#19306=EDGE_CURVE('',#15225,#15226,#9082,.T.);
#19307=EDGE_CURVE('',#15225,#15227,#9083,.T.);
#19308=EDGE_CURVE('',#15227,#15228,#9084,.T.);
#19309=EDGE_CURVE('',#15226,#15228,#9085,.T.);
#19310=EDGE_CURVE('',#15229,#15225,#9086,.T.);
#19311=EDGE_CURVE('',#15229,#15230,#9087,.T.);
#19312=EDGE_CURVE('',#15230,#15227,#9088,.T.);
#19313=EDGE_CURVE('',#15231,#15229,#9089,.T.);
#19314=EDGE_CURVE('',#15231,#15232,#9090,.T.);
#19315=EDGE_CURVE('',#15232,#15230,#9091,.T.);
#19316=EDGE_CURVE('',#15226,#15231,#9092,.T.);
#19317=EDGE_CURVE('',#15228,#15232,#9093,.T.);
#19318=EDGE_CURVE('',#15233,#15234,#9094,.T.);
#19319=EDGE_CURVE('',#15233,#15235,#9095,.T.);
#19320=EDGE_CURVE('',#15235,#15236,#9096,.T.);
#19321=EDGE_CURVE('',#15234,#15236,#9097,.T.);
#19322=EDGE_CURVE('',#15237,#15233,#9098,.T.);
#19323=EDGE_CURVE('',#15237,#15238,#9099,.T.);
#19324=EDGE_CURVE('',#15238,#15235,#9100,.T.);
#19325=EDGE_CURVE('',#15239,#15237,#9101,.T.);
#19326=EDGE_CURVE('',#15239,#15240,#9102,.T.);
#19327=EDGE_CURVE('',#15240,#15238,#9103,.T.);
#19328=EDGE_CURVE('',#15234,#15239,#9104,.T.);
#19329=EDGE_CURVE('',#15236,#15240,#9105,.T.);
#19330=EDGE_CURVE('',#15241,#15242,#9106,.T.);
#19331=EDGE_CURVE('',#15241,#15243,#9107,.T.);
#19332=EDGE_CURVE('',#15243,#15244,#9108,.T.);
#19333=EDGE_CURVE('',#15242,#15244,#9109,.T.);
#19334=EDGE_CURVE('',#15245,#15241,#9110,.T.);
#19335=EDGE_CURVE('',#15245,#15246,#9111,.T.);
#19336=EDGE_CURVE('',#15246,#15243,#9112,.T.);
#19337=EDGE_CURVE('',#15247,#15245,#9113,.T.);
#19338=EDGE_CURVE('',#15247,#15248,#9114,.T.);
#19339=EDGE_CURVE('',#15248,#15246,#9115,.T.);
#19340=EDGE_CURVE('',#15242,#15247,#9116,.T.);
#19341=EDGE_CURVE('',#15244,#15248,#9117,.T.);
#19342=EDGE_CURVE('',#15249,#15250,#9118,.T.);
#19343=EDGE_CURVE('',#15249,#15251,#9119,.T.);
#19344=EDGE_CURVE('',#15251,#15252,#9120,.T.);
#19345=EDGE_CURVE('',#15250,#15252,#9121,.T.);
#19346=EDGE_CURVE('',#15253,#15249,#9122,.T.);
#19347=EDGE_CURVE('',#15253,#15254,#9123,.T.);
#19348=EDGE_CURVE('',#15254,#15251,#9124,.T.);
#19349=EDGE_CURVE('',#15255,#15253,#9125,.T.);
#19350=EDGE_CURVE('',#15255,#15256,#9126,.T.);
#19351=EDGE_CURVE('',#15256,#15254,#9127,.T.);
#19352=EDGE_CURVE('',#15250,#15255,#9128,.T.);
#19353=EDGE_CURVE('',#15252,#15256,#9129,.T.);
#19354=EDGE_CURVE('',#15257,#15258,#9130,.T.);
#19355=EDGE_CURVE('',#15257,#15259,#9131,.T.);
#19356=EDGE_CURVE('',#15259,#15260,#9132,.T.);
#19357=EDGE_CURVE('',#15258,#15260,#9133,.T.);
#19358=EDGE_CURVE('',#15261,#15257,#9134,.T.);
#19359=EDGE_CURVE('',#15261,#15262,#9135,.T.);
#19360=EDGE_CURVE('',#15262,#15259,#9136,.T.);
#19361=EDGE_CURVE('',#15263,#15261,#9137,.T.);
#19362=EDGE_CURVE('',#15263,#15264,#9138,.T.);
#19363=EDGE_CURVE('',#15264,#15262,#9139,.T.);
#19364=EDGE_CURVE('',#15258,#15263,#9140,.T.);
#19365=EDGE_CURVE('',#15260,#15264,#9141,.T.);
#19366=EDGE_CURVE('',#15265,#15266,#9142,.T.);
#19367=EDGE_CURVE('',#15265,#15267,#9143,.T.);
#19368=EDGE_CURVE('',#15267,#15268,#9144,.T.);
#19369=EDGE_CURVE('',#15266,#15268,#9145,.T.);
#19370=EDGE_CURVE('',#15269,#15265,#9146,.T.);
#19371=EDGE_CURVE('',#15269,#15270,#9147,.T.);
#19372=EDGE_CURVE('',#15270,#15267,#9148,.T.);
#19373=EDGE_CURVE('',#15271,#15269,#9149,.T.);
#19374=EDGE_CURVE('',#15271,#15272,#9150,.T.);
#19375=EDGE_CURVE('',#15272,#15270,#9151,.T.);
#19376=EDGE_CURVE('',#15266,#15271,#9152,.T.);
#19377=EDGE_CURVE('',#15268,#15272,#9153,.T.);
#19378=EDGE_CURVE('',#15273,#15274,#9154,.T.);
#19379=EDGE_CURVE('',#15273,#15275,#9155,.T.);
#19380=EDGE_CURVE('',#15275,#15276,#9156,.T.);
#19381=EDGE_CURVE('',#15274,#15276,#9157,.T.);
#19382=EDGE_CURVE('',#15277,#15273,#9158,.T.);
#19383=EDGE_CURVE('',#15277,#15278,#9159,.T.);
#19384=EDGE_CURVE('',#15278,#15275,#9160,.T.);
#19385=EDGE_CURVE('',#15279,#15277,#9161,.T.);
#19386=EDGE_CURVE('',#15279,#15280,#9162,.T.);
#19387=EDGE_CURVE('',#15280,#15278,#9163,.T.);
#19388=EDGE_CURVE('',#15274,#15279,#9164,.T.);
#19389=EDGE_CURVE('',#15276,#15280,#9165,.T.);
#19390=EDGE_CURVE('',#15281,#15282,#9166,.T.);
#19391=EDGE_CURVE('',#15281,#15283,#9167,.T.);
#19392=EDGE_CURVE('',#15283,#15284,#9168,.T.);
#19393=EDGE_CURVE('',#15282,#15284,#9169,.T.);
#19394=EDGE_CURVE('',#15285,#15281,#9170,.T.);
#19395=EDGE_CURVE('',#15285,#15286,#9171,.T.);
#19396=EDGE_CURVE('',#15286,#15283,#9172,.T.);
#19397=EDGE_CURVE('',#15287,#15285,#9173,.T.);
#19398=EDGE_CURVE('',#15287,#15288,#9174,.T.);
#19399=EDGE_CURVE('',#15288,#15286,#9175,.T.);
#19400=EDGE_CURVE('',#15282,#15287,#9176,.T.);
#19401=EDGE_CURVE('',#15284,#15288,#9177,.T.);
#19402=EDGE_CURVE('',#15289,#15290,#9178,.T.);
#19403=EDGE_CURVE('',#15289,#15291,#9179,.T.);
#19404=EDGE_CURVE('',#15291,#15292,#9180,.T.);
#19405=EDGE_CURVE('',#15290,#15292,#9181,.T.);
#19406=EDGE_CURVE('',#15293,#15289,#9182,.T.);
#19407=EDGE_CURVE('',#15293,#15294,#9183,.T.);
#19408=EDGE_CURVE('',#15294,#15291,#9184,.T.);
#19409=EDGE_CURVE('',#15295,#15293,#9185,.T.);
#19410=EDGE_CURVE('',#15295,#15296,#9186,.T.);
#19411=EDGE_CURVE('',#15296,#15294,#9187,.T.);
#19412=EDGE_CURVE('',#15290,#15295,#9188,.T.);
#19413=EDGE_CURVE('',#15292,#15296,#9189,.T.);
#19414=EDGE_CURVE('',#15297,#15297,#12928,.T.);
#19415=EDGE_CURVE('',#15297,#15298,#9190,.T.);
#19416=EDGE_CURVE('',#15298,#15298,#12929,.T.);
#19417=EDGE_CURVE('',#15299,#15299,#12930,.T.);
#19418=EDGE_CURVE('',#15299,#15300,#9191,.T.);
#19419=EDGE_CURVE('',#15300,#15300,#12931,.T.);
#19420=EDGE_CURVE('',#15301,#15302,#9192,.T.);
#19421=EDGE_CURVE('',#15301,#15303,#9193,.T.);
#19422=EDGE_CURVE('',#15304,#15303,#9194,.T.);
#19423=EDGE_CURVE('',#15302,#15304,#9195,.T.);
#19424=EDGE_CURVE('',#15302,#15305,#9196,.T.);
#19425=EDGE_CURVE('',#15306,#15304,#9197,.T.);
#19426=EDGE_CURVE('',#15305,#15306,#9198,.T.);
#19427=EDGE_CURVE('',#15305,#15307,#9199,.T.);
#19428=EDGE_CURVE('',#15308,#15306,#9200,.T.);
#19429=EDGE_CURVE('',#15307,#15308,#9201,.T.);
#19430=EDGE_CURVE('',#15307,#15309,#9202,.T.);
#19431=EDGE_CURVE('',#15310,#15308,#9203,.T.);
#19432=EDGE_CURVE('',#15309,#15310,#9204,.T.);
#19433=EDGE_CURVE('',#15309,#15311,#9205,.T.);
#19434=EDGE_CURVE('',#15312,#15310,#9206,.T.);
#19435=EDGE_CURVE('',#15311,#15312,#9207,.T.);
#19436=EDGE_CURVE('',#15311,#15313,#9208,.T.);
#19437=EDGE_CURVE('',#15314,#15312,#9209,.T.);
#19438=EDGE_CURVE('',#15313,#15314,#9210,.T.);
#19439=EDGE_CURVE('',#15313,#15315,#9211,.T.);
#19440=EDGE_CURVE('',#15316,#15314,#9212,.T.);
#19441=EDGE_CURVE('',#15315,#15316,#9213,.T.);
#19442=EDGE_CURVE('',#15315,#15301,#9214,.T.);
#19443=EDGE_CURVE('',#15303,#15316,#9215,.T.);
#26862=ORIENTED_EDGE('',*,*,#19282,.F.);
#26863=ORIENTED_EDGE('',*,*,#19283,.T.);
#26864=ORIENTED_EDGE('',*,*,#19284,.T.);
#26865=ORIENTED_EDGE('',*,*,#19285,.F.);
#26866=ORIENTED_EDGE('',*,*,#19286,.F.);
#26867=ORIENTED_EDGE('',*,*,#19287,.T.);
#26868=ORIENTED_EDGE('',*,*,#19288,.T.);
#26869=ORIENTED_EDGE('',*,*,#19283,.F.);
#26870=ORIENTED_EDGE('',*,*,#19289,.F.);
#26871=ORIENTED_EDGE('',*,*,#19290,.T.);
#26872=ORIENTED_EDGE('',*,*,#19291,.T.);
#26873=ORIENTED_EDGE('',*,*,#19287,.F.);
#26874=ORIENTED_EDGE('',*,*,#19292,.F.);
#26875=ORIENTED_EDGE('',*,*,#19285,.T.);
#26876=ORIENTED_EDGE('',*,*,#19293,.T.);
#26877=ORIENTED_EDGE('',*,*,#19290,.F.);
#26878=ORIENTED_EDGE('',*,*,#19293,.F.);
#26879=ORIENTED_EDGE('',*,*,#19284,.F.);
#26880=ORIENTED_EDGE('',*,*,#19288,.F.);
#26881=ORIENTED_EDGE('',*,*,#19291,.F.);
#26882=ORIENTED_EDGE('',*,*,#19294,.F.);
#26883=ORIENTED_EDGE('',*,*,#19295,.T.);
#26884=ORIENTED_EDGE('',*,*,#19296,.T.);
#26885=ORIENTED_EDGE('',*,*,#19297,.F.);
#26886=ORIENTED_EDGE('',*,*,#19298,.F.);
#26887=ORIENTED_EDGE('',*,*,#19299,.T.);
#26888=ORIENTED_EDGE('',*,*,#19300,.T.);
#26889=ORIENTED_EDGE('',*,*,#19295,.F.);
#26890=ORIENTED_EDGE('',*,*,#19301,.F.);
#26891=ORIENTED_EDGE('',*,*,#19302,.T.);
#26892=ORIENTED_EDGE('',*,*,#19303,.T.);
#26893=ORIENTED_EDGE('',*,*,#19299,.F.);
#26894=ORIENTED_EDGE('',*,*,#19304,.F.);
#26895=ORIENTED_EDGE('',*,*,#19297,.T.);
#26896=ORIENTED_EDGE('',*,*,#19305,.T.);
#26897=ORIENTED_EDGE('',*,*,#19302,.F.);
#26898=ORIENTED_EDGE('',*,*,#19305,.F.);
#26899=ORIENTED_EDGE('',*,*,#19296,.F.);
#26900=ORIENTED_EDGE('',*,*,#19300,.F.);
#26901=ORIENTED_EDGE('',*,*,#19303,.F.);
#26902=ORIENTED_EDGE('',*,*,#19306,.F.);
#26903=ORIENTED_EDGE('',*,*,#19307,.T.);
#26904=ORIENTED_EDGE('',*,*,#19308,.T.);
#26905=ORIENTED_EDGE('',*,*,#19309,.F.);
#26906=ORIENTED_EDGE('',*,*,#19310,.F.);
#26907=ORIENTED_EDGE('',*,*,#19311,.T.);
#26908=ORIENTED_EDGE('',*,*,#19312,.T.);
#26909=ORIENTED_EDGE('',*,*,#19307,.F.);
#26910=ORIENTED_EDGE('',*,*,#19313,.F.);
#26911=ORIENTED_EDGE('',*,*,#19314,.T.);
#26912=ORIENTED_EDGE('',*,*,#19315,.T.);
#26913=ORIENTED_EDGE('',*,*,#19311,.F.);
#26914=ORIENTED_EDGE('',*,*,#19316,.F.);
#26915=ORIENTED_EDGE('',*,*,#19309,.T.);
#26916=ORIENTED_EDGE('',*,*,#19317,.T.);
#26917=ORIENTED_EDGE('',*,*,#19314,.F.);
#26918=ORIENTED_EDGE('',*,*,#19317,.F.);
#26919=ORIENTED_EDGE('',*,*,#19308,.F.);
#26920=ORIENTED_EDGE('',*,*,#19312,.F.);
#26921=ORIENTED_EDGE('',*,*,#19315,.F.);
#26922=ORIENTED_EDGE('',*,*,#19318,.F.);
#26923=ORIENTED_EDGE('',*,*,#19319,.T.);
#26924=ORIENTED_EDGE('',*,*,#19320,.T.);
#26925=ORIENTED_EDGE('',*,*,#19321,.F.);
#26926=ORIENTED_EDGE('',*,*,#19322,.F.);
#26927=ORIENTED_EDGE('',*,*,#19323,.T.);
#26928=ORIENTED_EDGE('',*,*,#19324,.T.);
#26929=ORIENTED_EDGE('',*,*,#19319,.F.);
#26930=ORIENTED_EDGE('',*,*,#19325,.F.);
#26931=ORIENTED_EDGE('',*,*,#19326,.T.);
#26932=ORIENTED_EDGE('',*,*,#19327,.T.);
#26933=ORIENTED_EDGE('',*,*,#19323,.F.);
#26934=ORIENTED_EDGE('',*,*,#19328,.F.);
#26935=ORIENTED_EDGE('',*,*,#19321,.T.);
#26936=ORIENTED_EDGE('',*,*,#19329,.T.);
#26937=ORIENTED_EDGE('',*,*,#19326,.F.);
#26938=ORIENTED_EDGE('',*,*,#19329,.F.);
#26939=ORIENTED_EDGE('',*,*,#19320,.F.);
#26940=ORIENTED_EDGE('',*,*,#19324,.F.);
#26941=ORIENTED_EDGE('',*,*,#19327,.F.);
#26942=ORIENTED_EDGE('',*,*,#19330,.F.);
#26943=ORIENTED_EDGE('',*,*,#19331,.T.);
#26944=ORIENTED_EDGE('',*,*,#19332,.T.);
#26945=ORIENTED_EDGE('',*,*,#19333,.F.);
#26946=ORIENTED_EDGE('',*,*,#19334,.F.);
#26947=ORIENTED_EDGE('',*,*,#19335,.T.);
#26948=ORIENTED_EDGE('',*,*,#19336,.T.);
#26949=ORIENTED_EDGE('',*,*,#19331,.F.);
#26950=ORIENTED_EDGE('',*,*,#19337,.F.);
#26951=ORIENTED_EDGE('',*,*,#19338,.T.);
#26952=ORIENTED_EDGE('',*,*,#19339,.T.);
#26953=ORIENTED_EDGE('',*,*,#19335,.F.);
#26954=ORIENTED_EDGE('',*,*,#19340,.F.);
#26955=ORIENTED_EDGE('',*,*,#19333,.T.);
#26956=ORIENTED_EDGE('',*,*,#19341,.T.);
#26957=ORIENTED_EDGE('',*,*,#19338,.F.);
#26958=ORIENTED_EDGE('',*,*,#19341,.F.);
#26959=ORIENTED_EDGE('',*,*,#19332,.F.);
#26960=ORIENTED_EDGE('',*,*,#19336,.F.);
#26961=ORIENTED_EDGE('',*,*,#19339,.F.);
#26962=ORIENTED_EDGE('',*,*,#19342,.F.);
#26963=ORIENTED_EDGE('',*,*,#19343,.T.);
#26964=ORIENTED_EDGE('',*,*,#19344,.T.);
#26965=ORIENTED_EDGE('',*,*,#19345,.F.);
#26966=ORIENTED_EDGE('',*,*,#19346,.F.);
#26967=ORIENTED_EDGE('',*,*,#19347,.T.);
#26968=ORIENTED_EDGE('',*,*,#19348,.T.);
#26969=ORIENTED_EDGE('',*,*,#19343,.F.);
#26970=ORIENTED_EDGE('',*,*,#19349,.F.);
#26971=ORIENTED_EDGE('',*,*,#19350,.T.);
#26972=ORIENTED_EDGE('',*,*,#19351,.T.);
#26973=ORIENTED_EDGE('',*,*,#19347,.F.);
#26974=ORIENTED_EDGE('',*,*,#19352,.F.);
#26975=ORIENTED_EDGE('',*,*,#19345,.T.);
#26976=ORIENTED_EDGE('',*,*,#19353,.T.);
#26977=ORIENTED_EDGE('',*,*,#19350,.F.);
#26978=ORIENTED_EDGE('',*,*,#19353,.F.);
#26979=ORIENTED_EDGE('',*,*,#19344,.F.);
#26980=ORIENTED_EDGE('',*,*,#19348,.F.);
#26981=ORIENTED_EDGE('',*,*,#19351,.F.);
#26982=ORIENTED_EDGE('',*,*,#19354,.F.);
#26983=ORIENTED_EDGE('',*,*,#19355,.T.);
#26984=ORIENTED_EDGE('',*,*,#19356,.T.);
#26985=ORIENTED_EDGE('',*,*,#19357,.F.);
#26986=ORIENTED_EDGE('',*,*,#19358,.F.);
#26987=ORIENTED_EDGE('',*,*,#19359,.T.);
#26988=ORIENTED_EDGE('',*,*,#19360,.T.);
#26989=ORIENTED_EDGE('',*,*,#19355,.F.);
#26990=ORIENTED_EDGE('',*,*,#19361,.F.);
#26991=ORIENTED_EDGE('',*,*,#19362,.T.);
#26992=ORIENTED_EDGE('',*,*,#19363,.T.);
#26993=ORIENTED_EDGE('',*,*,#19359,.F.);
#26994=ORIENTED_EDGE('',*,*,#19364,.F.);
#26995=ORIENTED_EDGE('',*,*,#19357,.T.);
#26996=ORIENTED_EDGE('',*,*,#19365,.T.);
#26997=ORIENTED_EDGE('',*,*,#19362,.F.);
#26998=ORIENTED_EDGE('',*,*,#19365,.F.);
#26999=ORIENTED_EDGE('',*,*,#19356,.F.);
#27000=ORIENTED_EDGE('',*,*,#19360,.F.);
#27001=ORIENTED_EDGE('',*,*,#19363,.F.);
#27002=ORIENTED_EDGE('',*,*,#19366,.F.);
#27003=ORIENTED_EDGE('',*,*,#19367,.T.);
#27004=ORIENTED_EDGE('',*,*,#19368,.T.);
#27005=ORIENTED_EDGE('',*,*,#19369,.F.);
#27006=ORIENTED_EDGE('',*,*,#19370,.F.);
#27007=ORIENTED_EDGE('',*,*,#19371,.T.);
#27008=ORIENTED_EDGE('',*,*,#19372,.T.);
#27009=ORIENTED_EDGE('',*,*,#19367,.F.);
#27010=ORIENTED_EDGE('',*,*,#19373,.F.);
#27011=ORIENTED_EDGE('',*,*,#19374,.T.);
#27012=ORIENTED_EDGE('',*,*,#19375,.T.);
#27013=ORIENTED_EDGE('',*,*,#19371,.F.);
#27014=ORIENTED_EDGE('',*,*,#19376,.F.);
#27015=ORIENTED_EDGE('',*,*,#19369,.T.);
#27016=ORIENTED_EDGE('',*,*,#19377,.T.);
#27017=ORIENTED_EDGE('',*,*,#19374,.F.);
#27018=ORIENTED_EDGE('',*,*,#19377,.F.);
#27019=ORIENTED_EDGE('',*,*,#19368,.F.);
#27020=ORIENTED_EDGE('',*,*,#19372,.F.);
#27021=ORIENTED_EDGE('',*,*,#19375,.F.);
#27022=ORIENTED_EDGE('',*,*,#19378,.F.);
#27023=ORIENTED_EDGE('',*,*,#19379,.T.);
#27024=ORIENTED_EDGE('',*,*,#19380,.T.);
#27025=ORIENTED_EDGE('',*,*,#19381,.F.);
#27026=ORIENTED_EDGE('',*,*,#19382,.F.);
#27027=ORIENTED_EDGE('',*,*,#19383,.T.);
#27028=ORIENTED_EDGE('',*,*,#19384,.T.);
#27029=ORIENTED_EDGE('',*,*,#19379,.F.);
#27030=ORIENTED_EDGE('',*,*,#19385,.F.);
#27031=ORIENTED_EDGE('',*,*,#19386,.T.);
#27032=ORIENTED_EDGE('',*,*,#19387,.T.);
#27033=ORIENTED_EDGE('',*,*,#19383,.F.);
#27034=ORIENTED_EDGE('',*,*,#19388,.F.);
#27035=ORIENTED_EDGE('',*,*,#19381,.T.);
#27036=ORIENTED_EDGE('',*,*,#19389,.T.);
#27037=ORIENTED_EDGE('',*,*,#19386,.F.);
#27038=ORIENTED_EDGE('',*,*,#19389,.F.);
#27039=ORIENTED_EDGE('',*,*,#19380,.F.);
#27040=ORIENTED_EDGE('',*,*,#19384,.F.);
#27041=ORIENTED_EDGE('',*,*,#19387,.F.);
#27042=ORIENTED_EDGE('',*,*,#19390,.F.);
#27043=ORIENTED_EDGE('',*,*,#19391,.T.);
#27044=ORIENTED_EDGE('',*,*,#19392,.T.);
#27045=ORIENTED_EDGE('',*,*,#19393,.F.);
#27046=ORIENTED_EDGE('',*,*,#19394,.F.);
#27047=ORIENTED_EDGE('',*,*,#19395,.T.);
#27048=ORIENTED_EDGE('',*,*,#19396,.T.);
#27049=ORIENTED_EDGE('',*,*,#19391,.F.);
#27050=ORIENTED_EDGE('',*,*,#19397,.F.);
#27051=ORIENTED_EDGE('',*,*,#19398,.T.);
#27052=ORIENTED_EDGE('',*,*,#19399,.T.);
#27053=ORIENTED_EDGE('',*,*,#19395,.F.);
#27054=ORIENTED_EDGE('',*,*,#19400,.F.);
#27055=ORIENTED_EDGE('',*,*,#19393,.T.);
#27056=ORIENTED_EDGE('',*,*,#19401,.T.);
#27057=ORIENTED_EDGE('',*,*,#19398,.F.);
#27058=ORIENTED_EDGE('',*,*,#19401,.F.);
#27059=ORIENTED_EDGE('',*,*,#19392,.F.);
#27060=ORIENTED_EDGE('',*,*,#19396,.F.);
#27061=ORIENTED_EDGE('',*,*,#19399,.F.);
#27062=ORIENTED_EDGE('',*,*,#19402,.F.);
#27063=ORIENTED_EDGE('',*,*,#19403,.T.);
#27064=ORIENTED_EDGE('',*,*,#19404,.T.);
#27065=ORIENTED_EDGE('',*,*,#19405,.F.);
#27066=ORIENTED_EDGE('',*,*,#19406,.F.);
#27067=ORIENTED_EDGE('',*,*,#19407,.T.);
#27068=ORIENTED_EDGE('',*,*,#19408,.T.);
#27069=ORIENTED_EDGE('',*,*,#19403,.F.);
#27070=ORIENTED_EDGE('',*,*,#19409,.F.);
#27071=ORIENTED_EDGE('',*,*,#19410,.T.);
#27072=ORIENTED_EDGE('',*,*,#19411,.T.);
#27073=ORIENTED_EDGE('',*,*,#19407,.F.);
#27074=ORIENTED_EDGE('',*,*,#19412,.F.);
#27075=ORIENTED_EDGE('',*,*,#19405,.T.);
#27076=ORIENTED_EDGE('',*,*,#19413,.T.);
#27077=ORIENTED_EDGE('',*,*,#19410,.F.);
#27078=ORIENTED_EDGE('',*,*,#19413,.F.);
#27079=ORIENTED_EDGE('',*,*,#19404,.F.);
#27080=ORIENTED_EDGE('',*,*,#19408,.F.);
#27081=ORIENTED_EDGE('',*,*,#19411,.F.);
#27082=ORIENTED_EDGE('',*,*,#19414,.F.);
#27083=ORIENTED_EDGE('',*,*,#19415,.T.);
#27084=ORIENTED_EDGE('',*,*,#19416,.F.);
#27085=ORIENTED_EDGE('',*,*,#19415,.F.);
#27086=ORIENTED_EDGE('',*,*,#19417,.F.);
#27087=ORIENTED_EDGE('',*,*,#19418,.T.);
#27088=ORIENTED_EDGE('',*,*,#19419,.F.);
#27089=ORIENTED_EDGE('',*,*,#19418,.F.);
#27090=ORIENTED_EDGE('',*,*,#19420,.F.);
#27091=ORIENTED_EDGE('',*,*,#19421,.T.);
#27092=ORIENTED_EDGE('',*,*,#19422,.F.);
#27093=ORIENTED_EDGE('',*,*,#19423,.F.);
#27094=ORIENTED_EDGE('',*,*,#19414,.T.);
#27095=ORIENTED_EDGE('',*,*,#19417,.T.);
#27096=ORIENTED_EDGE('',*,*,#19424,.F.);
#27097=ORIENTED_EDGE('',*,*,#19423,.T.);
#27098=ORIENTED_EDGE('',*,*,#19425,.F.);
#27099=ORIENTED_EDGE('',*,*,#19426,.F.);
#27100=ORIENTED_EDGE('',*,*,#19427,.F.);
#27101=ORIENTED_EDGE('',*,*,#19426,.T.);
#27102=ORIENTED_EDGE('',*,*,#19428,.F.);
#27103=ORIENTED_EDGE('',*,*,#19429,.F.);
#27104=ORIENTED_EDGE('',*,*,#19416,.T.);
#27105=ORIENTED_EDGE('',*,*,#19419,.T.);
#27106=ORIENTED_EDGE('',*,*,#19430,.F.);
#27107=ORIENTED_EDGE('',*,*,#19429,.T.);
#27108=ORIENTED_EDGE('',*,*,#19431,.F.);
#27109=ORIENTED_EDGE('',*,*,#19432,.F.);
#27110=ORIENTED_EDGE('',*,*,#19433,.F.);
#27111=ORIENTED_EDGE('',*,*,#19432,.T.);
#27112=ORIENTED_EDGE('',*,*,#19434,.F.);
#27113=ORIENTED_EDGE('',*,*,#19435,.F.);
#27114=ORIENTED_EDGE('',*,*,#19436,.F.);
#27115=ORIENTED_EDGE('',*,*,#19435,.T.);
#27116=ORIENTED_EDGE('',*,*,#19437,.F.);
#27117=ORIENTED_EDGE('',*,*,#19438,.F.);
#27118=ORIENTED_EDGE('',*,*,#19439,.F.);
#27119=ORIENTED_EDGE('',*,*,#19438,.T.);
#27120=ORIENTED_EDGE('',*,*,#19440,.F.);
#27121=ORIENTED_EDGE('',*,*,#19441,.F.);
#27122=ORIENTED_EDGE('',*,*,#19402,.T.);
#27123=ORIENTED_EDGE('',*,*,#19412,.T.);
#27124=ORIENTED_EDGE('',*,*,#19409,.T.);
#27125=ORIENTED_EDGE('',*,*,#19406,.T.);
#27126=ORIENTED_EDGE('',*,*,#19390,.T.);
#27127=ORIENTED_EDGE('',*,*,#19400,.T.);
#27128=ORIENTED_EDGE('',*,*,#19397,.T.);
#27129=ORIENTED_EDGE('',*,*,#19394,.T.);
#27130=ORIENTED_EDGE('',*,*,#19378,.T.);
#27131=ORIENTED_EDGE('',*,*,#19388,.T.);
#27132=ORIENTED_EDGE('',*,*,#19385,.T.);
#27133=ORIENTED_EDGE('',*,*,#19382,.T.);
#27134=ORIENTED_EDGE('',*,*,#19366,.T.);
#27135=ORIENTED_EDGE('',*,*,#19376,.T.);
#27136=ORIENTED_EDGE('',*,*,#19373,.T.);
#27137=ORIENTED_EDGE('',*,*,#19370,.T.);
#27138=ORIENTED_EDGE('',*,*,#19354,.T.);
#27139=ORIENTED_EDGE('',*,*,#19364,.T.);
#27140=ORIENTED_EDGE('',*,*,#19361,.T.);
#27141=ORIENTED_EDGE('',*,*,#19358,.T.);
#27142=ORIENTED_EDGE('',*,*,#19342,.T.);
#27143=ORIENTED_EDGE('',*,*,#19352,.T.);
#27144=ORIENTED_EDGE('',*,*,#19349,.T.);
#27145=ORIENTED_EDGE('',*,*,#19346,.T.);
#27146=ORIENTED_EDGE('',*,*,#19330,.T.);
#27147=ORIENTED_EDGE('',*,*,#19340,.T.);
#27148=ORIENTED_EDGE('',*,*,#19337,.T.);
#27149=ORIENTED_EDGE('',*,*,#19334,.T.);
#27150=ORIENTED_EDGE('',*,*,#19318,.T.);
#27151=ORIENTED_EDGE('',*,*,#19328,.T.);
#27152=ORIENTED_EDGE('',*,*,#19325,.T.);
#27153=ORIENTED_EDGE('',*,*,#19322,.T.);
#27154=ORIENTED_EDGE('',*,*,#19306,.T.);
#27155=ORIENTED_EDGE('',*,*,#19316,.T.);
#27156=ORIENTED_EDGE('',*,*,#19313,.T.);
#27157=ORIENTED_EDGE('',*,*,#19310,.T.);
#27158=ORIENTED_EDGE('',*,*,#19294,.T.);
#27159=ORIENTED_EDGE('',*,*,#19304,.T.);
#27160=ORIENTED_EDGE('',*,*,#19301,.T.);
#27161=ORIENTED_EDGE('',*,*,#19298,.T.);
#27162=ORIENTED_EDGE('',*,*,#19282,.T.);
#27163=ORIENTED_EDGE('',*,*,#19292,.T.);
#27164=ORIENTED_EDGE('',*,*,#19289,.T.);
#27165=ORIENTED_EDGE('',*,*,#19286,.T.);
#27166=ORIENTED_EDGE('',*,*,#19442,.F.);
#27167=ORIENTED_EDGE('',*,*,#19441,.T.);
#27168=ORIENTED_EDGE('',*,*,#19443,.F.);
#27169=ORIENTED_EDGE('',*,*,#19421,.F.);
#27170=ORIENTED_EDGE('',*,*,#19443,.T.);
#27171=ORIENTED_EDGE('',*,*,#19440,.T.);
#27172=ORIENTED_EDGE('',*,*,#19437,.T.);
#27173=ORIENTED_EDGE('',*,*,#19434,.T.);
#27174=ORIENTED_EDGE('',*,*,#19431,.T.);
#27175=ORIENTED_EDGE('',*,*,#19428,.T.);
#27176=ORIENTED_EDGE('',*,*,#19425,.T.);
#27177=ORIENTED_EDGE('',*,*,#19422,.T.);
#27178=ORIENTED_EDGE('',*,*,#19442,.T.);
#27179=ORIENTED_EDGE('',*,*,#19420,.T.);
#27180=ORIENTED_EDGE('',*,*,#19424,.T.);
#27181=ORIENTED_EDGE('',*,*,#19427,.T.);
#27182=ORIENTED_EDGE('',*,*,#19430,.T.);
#27183=ORIENTED_EDGE('',*,*,#19433,.T.);
#27184=ORIENTED_EDGE('',*,*,#19436,.T.);
#27185=ORIENTED_EDGE('',*,*,#19439,.T.);
#31478=ADVANCED_FACE('',(#4503),#2961,.F.);
#31479=ADVANCED_FACE('',(#4504),#2962,.F.);
#31480=ADVANCED_FACE('',(#4505),#2963,.F.);
#31481=ADVANCED_FACE('',(#4506),#2964,.F.);
#31482=ADVANCED_FACE('',(#4507),#2965,.F.);
#31483=ADVANCED_FACE('',(#4508),#2966,.F.);
#31484=ADVANCED_FACE('',(#4509),#2967,.F.);
#31485=ADVANCED_FACE('',(#4510),#2968,.F.);
#31486=ADVANCED_FACE('',(#4511),#2969,.F.);
#31487=ADVANCED_FACE('',(#4512),#2970,.F.);
#31488=ADVANCED_FACE('',(#4513),#2971,.F.);
#31489=ADVANCED_FACE('',(#4514),#2972,.F.);
#31490=ADVANCED_FACE('',(#4515),#2973,.F.);
#31491=ADVANCED_FACE('',(#4516),#2974,.F.);
#31492=ADVANCED_FACE('',(#4517),#2975,.F.);
#31493=ADVANCED_FACE('',(#4518),#2976,.F.);
#31494=ADVANCED_FACE('',(#4519),#2977,.F.);
#31495=ADVANCED_FACE('',(#4520),#2978,.F.);
#31496=ADVANCED_FACE('',(#4521),#2979,.F.);
#31497=ADVANCED_FACE('',(#4522),#2980,.F.);
#31498=ADVANCED_FACE('',(#4523),#2981,.F.);
#31499=ADVANCED_FACE('',(#4524),#2982,.F.);
#31500=ADVANCED_FACE('',(#4525),#2983,.F.);
#31501=ADVANCED_FACE('',(#4526),#2984,.F.);
#31502=ADVANCED_FACE('',(#4527),#2985,.F.);
#31503=ADVANCED_FACE('',(#4528),#2986,.F.);
#31504=ADVANCED_FACE('',(#4529),#2987,.F.);
#31505=ADVANCED_FACE('',(#4530),#2988,.F.);
#31506=ADVANCED_FACE('',(#4531),#2989,.F.);
#31507=ADVANCED_FACE('',(#4532),#2990,.F.);
#31508=ADVANCED_FACE('',(#4533),#2991,.F.);
#31509=ADVANCED_FACE('',(#4534),#2992,.F.);
#31510=ADVANCED_FACE('',(#4535),#2993,.F.);
#31511=ADVANCED_FACE('',(#4536),#2994,.F.);
#31512=ADVANCED_FACE('',(#4537),#2995,.F.);
#31513=ADVANCED_FACE('',(#4538),#2996,.F.);
#31514=ADVANCED_FACE('',(#4539),#2997,.F.);
#31515=ADVANCED_FACE('',(#4540),#2998,.F.);
#31516=ADVANCED_FACE('',(#4541),#2999,.F.);
#31517=ADVANCED_FACE('',(#4542),#3000,.F.);
#31518=ADVANCED_FACE('',(#4543),#3001,.F.);
#31519=ADVANCED_FACE('',(#4544),#3002,.F.);
#31520=ADVANCED_FACE('',(#4545),#3003,.F.);
#31521=ADVANCED_FACE('',(#4546),#3004,.F.);
#31522=ADVANCED_FACE('',(#4547),#3005,.F.);
#31523=ADVANCED_FACE('',(#4548),#3006,.F.);
#31524=ADVANCED_FACE('',(#4549),#3007,.F.);
#31525=ADVANCED_FACE('',(#4550),#3008,.F.);
#31526=ADVANCED_FACE('',(#4551),#3009,.F.);
#31527=ADVANCED_FACE('',(#4552),#3010,.F.);
#31528=ADVANCED_FACE('',(#4553),#3011,.F.);
#31529=ADVANCED_FACE('',(#4554),#3012,.F.);
#31530=ADVANCED_FACE('',(#4555),#3013,.F.);
#31531=ADVANCED_FACE('',(#4556),#3014,.F.);
#31532=ADVANCED_FACE('',(#4557),#3015,.F.);
#31533=ADVANCED_FACE('',(#4558),#1846,.F.);
#31534=ADVANCED_FACE('',(#4559),#1847,.F.);
#31535=ADVANCED_FACE('',(#4560,#2195,#2196),#3016,.T.);
#31536=ADVANCED_FACE('',(#4561),#3017,.T.);
#31537=ADVANCED_FACE('',(#4562,#2197,#2198),#3018,.T.);
#31538=ADVANCED_FACE('',(#4563),#3019,.T.);
#31539=ADVANCED_FACE('',(#4564),#3020,.T.);
#31540=ADVANCED_FACE('',(#4565),#3021,.T.);
#31541=ADVANCED_FACE('',(#4566,#2199,#2200,#2201,#2202,#2203,#2204,#2205,
#2206,#2207,#2208,#2209),#3022,.T.);
#31542=ADVANCED_FACE('',(#4567),#3023,.T.);
#31543=ADVANCED_FACE('',(#4568),#3024,.T.);
#31544=ADVANCED_FACE('',(#4569),#3025,.F.);
#32081=CLOSED_SHELL('',(#31478,#31479,#31480,#31481,#31482,#31483,#31484,
#31485,#31486,#31487,#31488,#31489,#31490,#31491,#31492,#31493,#31494,#31495,
#31496,#31497,#31498,#31499,#31500,#31501,#31502,#31503,#31504,#31505,#31506,
#31507,#31508,#31509,#31510,#31511,#31512,#31513,#31514,#31515,#31516,#31517,
#31518,#31519,#31520,#31521,#31522,#31523,#31524,#31525,#31526,#31527,#31528,
#31529,#31530,#31531,#31532,#31533,#31534,#31535,#31536,#31537,#31538,#31539,
#31540,#31541,#31542,#31543,#31544));
#33287=AXIS2_PLACEMENT_3D('',#76648,#38322,#38323);
#33288=AXIS2_PLACEMENT_3D('',#76649,#38324,#38325);
#33289=AXIS2_PLACEMENT_3D('',#76658,#38330,#38331);
#33290=AXIS2_PLACEMENT_3D('',#76664,#38335,#38336);
#33291=AXIS2_PLACEMENT_3D('',#76670,#38340,#38341);
#33292=AXIS2_PLACEMENT_3D('',#76673,#38344,#38345);
#33293=AXIS2_PLACEMENT_3D('',#76674,#38346,#38347);
#33294=AXIS2_PLACEMENT_3D('',#76683,#38352,#38353);
#33295=AXIS2_PLACEMENT_3D('',#76689,#38357,#38358);
#33296=AXIS2_PLACEMENT_3D('',#76695,#38362,#38363);
#33297=AXIS2_PLACEMENT_3D('',#76698,#38366,#38367);
#33298=AXIS2_PLACEMENT_3D('',#76699,#38368,#38369);
#33299=AXIS2_PLACEMENT_3D('',#76708,#38374,#38375);
#33300=AXIS2_PLACEMENT_3D('',#76714,#38379,#38380);
#33301=AXIS2_PLACEMENT_3D('',#76720,#38384,#38385);
#33302=AXIS2_PLACEMENT_3D('',#76723,#38388,#38389);
#33303=AXIS2_PLACEMENT_3D('',#76724,#38390,#38391);
#33304=AXIS2_PLACEMENT_3D('',#76733,#38396,#38397);
#33305=AXIS2_PLACEMENT_3D('',#76739,#38401,#38402);
#33306=AXIS2_PLACEMENT_3D('',#76745,#38406,#38407);
#33307=AXIS2_PLACEMENT_3D('',#76748,#38410,#38411);
#33308=AXIS2_PLACEMENT_3D('',#76749,#38412,#38413);
#33309=AXIS2_PLACEMENT_3D('',#76758,#38418,#38419);
#33310=AXIS2_PLACEMENT_3D('',#76764,#38423,#38424);
#33311=AXIS2_PLACEMENT_3D('',#76770,#38428,#38429);
#33312=AXIS2_PLACEMENT_3D('',#76773,#38432,#38433);
#33313=AXIS2_PLACEMENT_3D('',#76774,#38434,#38435);
#33314=AXIS2_PLACEMENT_3D('',#76783,#38440,#38441);
#33315=AXIS2_PLACEMENT_3D('',#76789,#38445,#38446);
#33316=AXIS2_PLACEMENT_3D('',#76795,#38450,#38451);
#33317=AXIS2_PLACEMENT_3D('',#76798,#38454,#38455);
#33318=AXIS2_PLACEMENT_3D('',#76799,#38456,#38457);
#33319=AXIS2_PLACEMENT_3D('',#76808,#38462,#38463);
#33320=AXIS2_PLACEMENT_3D('',#76814,#38467,#38468);
#33321=AXIS2_PLACEMENT_3D('',#76820,#38472,#38473);
#33322=AXIS2_PLACEMENT_3D('',#76823,#38476,#38477);
#33323=AXIS2_PLACEMENT_3D('',#76824,#38478,#38479);
#33324=AXIS2_PLACEMENT_3D('',#76833,#38484,#38485);
#33325=AXIS2_PLACEMENT_3D('',#76839,#38489,#38490);
#33326=AXIS2_PLACEMENT_3D('',#76845,#38494,#38495);
#33327=AXIS2_PLACEMENT_3D('',#76848,#38498,#38499);
#33328=AXIS2_PLACEMENT_3D('',#76849,#38500,#38501);
#33329=AXIS2_PLACEMENT_3D('',#76858,#38506,#38507);
#33330=AXIS2_PLACEMENT_3D('',#76864,#38511,#38512);
#33331=AXIS2_PLACEMENT_3D('',#76870,#38516,#38517);
#33332=AXIS2_PLACEMENT_3D('',#76873,#38520,#38521);
#33333=AXIS2_PLACEMENT_3D('',#76874,#38522,#38523);
#33334=AXIS2_PLACEMENT_3D('',#76883,#38528,#38529);
#33335=AXIS2_PLACEMENT_3D('',#76889,#38533,#38534);
#33336=AXIS2_PLACEMENT_3D('',#76895,#38538,#38539);
#33337=AXIS2_PLACEMENT_3D('',#76898,#38542,#38543);
#33338=AXIS2_PLACEMENT_3D('',#76899,#38544,#38545);
#33339=AXIS2_PLACEMENT_3D('',#76908,#38550,#38551);
#33340=AXIS2_PLACEMENT_3D('',#76914,#38555,#38556);
#33341=AXIS2_PLACEMENT_3D('',#76920,#38560,#38561);
#33342=AXIS2_PLACEMENT_3D('',#76923,#38564,#38565);
#33343=AXIS2_PLACEMENT_3D('',#76924,#38566,#38567);
#33344=AXIS2_PLACEMENT_3D('',#76926,#38568,#38569);
#33345=AXIS2_PLACEMENT_3D('',#76929,#38571,#38572);
#33346=AXIS2_PLACEMENT_3D('',#76930,#38573,#38574);
#33347=AXIS2_PLACEMENT_3D('',#76932,#38575,#38576);
#33348=AXIS2_PLACEMENT_3D('',#76935,#38578,#38579);
#33349=AXIS2_PLACEMENT_3D('',#76936,#38580,#38581);
#33350=AXIS2_PLACEMENT_3D('',#76945,#38586,#38587);
#33351=AXIS2_PLACEMENT_3D('',#76951,#38591,#38592);
#33352=AXIS2_PLACEMENT_3D('',#76957,#38596,#38597);
#33353=AXIS2_PLACEMENT_3D('',#76963,#38601,#38602);
#33354=AXIS2_PLACEMENT_3D('',#76969,#38606,#38607);
#33355=AXIS2_PLACEMENT_3D('',#76975,#38611,#38612);
#33356=AXIS2_PLACEMENT_3D('',#76981,#38616,#38617);
#33357=AXIS2_PLACEMENT_3D('',#76984,#38620,#38621);
#33358=AXIS2_PLACEMENT_3D('',#76985,#38622,#38623);
#38322=DIRECTION('axis',(0.,0.,1.));
#38323=DIRECTION('refdir',(1.,0.,0.));
#38324=DIRECTION('center_axis',(0.,0.,-1.));
#38325=DIRECTION('ref_axis',(0.,-1.,0.));
#38326=DIRECTION('',(0.,-1.,0.));
#38327=DIRECTION('',(-1.,0.,0.));
#38328=DIRECTION('',(0.,-1.,0.));
#38329=DIRECTION('',(-1.,0.,0.));
#38330=DIRECTION('center_axis',(0.,1.,0.));
#38331=DIRECTION('ref_axis',(0.,0.,-1.));
#38332=DIRECTION('',(0.,0.,-1.));
#38333=DIRECTION('',(-1.,0.,0.));
#38334=DIRECTION('',(0.,0.,-1.));
#38335=DIRECTION('center_axis',(0.,0.,1.));
#38336=DIRECTION('ref_axis',(0.,1.,0.));
#38337=DIRECTION('',(0.,1.,0.));
#38338=DIRECTION('',(-1.,0.,0.));
#38339=DIRECTION('',(0.,1.,0.));
#38340=DIRECTION('center_axis',(0.,-1.,0.));
#38341=DIRECTION('ref_axis',(0.,0.,1.));
#38342=DIRECTION('',(0.,0.,1.));
#38343=DIRECTION('',(0.,0.,1.));
#38344=DIRECTION('center_axis',(-1.,0.,0.));
#38345=DIRECTION('ref_axis',(0.,0.,1.));
#38346=DIRECTION('center_axis',(0.,0.,-1.));
#38347=DIRECTION('ref_axis',(0.,-1.,0.));
#38348=DIRECTION('',(0.,-1.,0.));
#38349=DIRECTION('',(-1.,0.,0.));
#38350=DIRECTION('',(0.,-1.,0.));
#38351=DIRECTION('',(-1.,0.,0.));
#38352=DIRECTION('center_axis',(0.,1.,0.));
#38353=DIRECTION('ref_axis',(0.,0.,-1.));
#38354=DIRECTION('',(0.,0.,-1.));
#38355=DIRECTION('',(-1.,0.,0.));
#38356=DIRECTION('',(0.,0.,-1.));
#38357=DIRECTION('center_axis',(0.,0.,1.));
#38358=DIRECTION('ref_axis',(0.,1.,0.));
#38359=DIRECTION('',(0.,1.,0.));
#38360=DIRECTION('',(-1.,0.,0.));
#38361=DIRECTION('',(0.,1.,0.));
#38362=DIRECTION('center_axis',(0.,-1.,0.));
#38363=DIRECTION('ref_axis',(0.,0.,1.));
#38364=DIRECTION('',(0.,0.,1.));
#38365=DIRECTION('',(0.,0.,1.));
#38366=DIRECTION('center_axis',(-1.,0.,0.));
#38367=DIRECTION('ref_axis',(0.,0.,1.));
#38368=DIRECTION('center_axis',(0.,0.,-1.));
#38369=DIRECTION('ref_axis',(0.,-1.,0.));
#38370=DIRECTION('',(0.,-1.,0.));
#38371=DIRECTION('',(-1.,0.,0.));
#38372=DIRECTION('',(0.,-1.,0.));
#38373=DIRECTION('',(-1.,0.,0.));
#38374=DIRECTION('center_axis',(0.,1.,0.));
#38375=DIRECTION('ref_axis',(0.,0.,-1.));
#38376=DIRECTION('',(0.,0.,-1.));
#38377=DIRECTION('',(-1.,0.,0.));
#38378=DIRECTION('',(0.,0.,-1.));
#38379=DIRECTION('center_axis',(0.,0.,1.));
#38380=DIRECTION('ref_axis',(0.,1.,0.));
#38381=DIRECTION('',(0.,1.,0.));
#38382=DIRECTION('',(-1.,0.,0.));
#38383=DIRECTION('',(0.,1.,0.));
#38384=DIRECTION('center_axis',(0.,-1.,0.));
#38385=DIRECTION('ref_axis',(0.,0.,1.));
#38386=DIRECTION('',(0.,0.,1.));
#38387=DIRECTION('',(0.,0.,1.));
#38388=DIRECTION('center_axis',(-1.,0.,0.));
#38389=DIRECTION('ref_axis',(0.,0.,1.));
#38390=DIRECTION('center_axis',(0.,0.,-1.));
#38391=DIRECTION('ref_axis',(0.,-1.,0.));
#38392=DIRECTION('',(0.,-1.,0.));
#38393=DIRECTION('',(-1.,0.,0.));
#38394=DIRECTION('',(0.,-1.,0.));
#38395=DIRECTION('',(-1.,0.,0.));
#38396=DIRECTION('center_axis',(0.,1.,0.));
#38397=DIRECTION('ref_axis',(0.,0.,-1.));
#38398=DIRECTION('',(0.,0.,-1.));
#38399=DIRECTION('',(-1.,0.,0.));
#38400=DIRECTION('',(0.,0.,-1.));
#38401=DIRECTION('center_axis',(0.,0.,1.));
#38402=DIRECTION('ref_axis',(0.,1.,0.));
#38403=DIRECTION('',(0.,1.,0.));
#38404=DIRECTION('',(-1.,0.,0.));
#38405=DIRECTION('',(0.,1.,0.));
#38406=DIRECTION('center_axis',(0.,-1.,0.));
#38407=DIRECTION('ref_axis',(0.,0.,1.));
#38408=DIRECTION('',(0.,0.,1.));
#38409=DIRECTION('',(0.,0.,1.));
#38410=DIRECTION('center_axis',(-1.,0.,0.));
#38411=DIRECTION('ref_axis',(0.,0.,1.));
#38412=DIRECTION('center_axis',(0.,0.,-1.));
#38413=DIRECTION('ref_axis',(0.,-1.,0.));
#38414=DIRECTION('',(0.,-1.,0.));
#38415=DIRECTION('',(-1.,0.,0.));
#38416=DIRECTION('',(0.,-1.,0.));
#38417=DIRECTION('',(-1.,0.,0.));
#38418=DIRECTION('center_axis',(0.,1.,0.));
#38419=DIRECTION('ref_axis',(0.,0.,-1.));
#38420=DIRECTION('',(0.,0.,-1.));
#38421=DIRECTION('',(-1.,0.,0.));
#38422=DIRECTION('',(0.,0.,-1.));
#38423=DIRECTION('center_axis',(0.,0.,1.));
#38424=DIRECTION('ref_axis',(0.,1.,0.));
#38425=DIRECTION('',(0.,1.,0.));
#38426=DIRECTION('',(-1.,0.,0.));
#38427=DIRECTION('',(0.,1.,0.));
#38428=DIRECTION('center_axis',(0.,-1.,0.));
#38429=DIRECTION('ref_axis',(0.,0.,1.));
#38430=DIRECTION('',(0.,0.,1.));
#38431=DIRECTION('',(0.,0.,1.));
#38432=DIRECTION('center_axis',(-1.,0.,0.));
#38433=DIRECTION('ref_axis',(0.,0.,1.));
#38434=DIRECTION('center_axis',(0.,0.,-1.));
#38435=DIRECTION('ref_axis',(0.,-1.,0.));
#38436=DIRECTION('',(0.,-1.,0.));
#38437=DIRECTION('',(-1.,0.,0.));
#38438=DIRECTION('',(0.,-1.,0.));
#38439=DIRECTION('',(-1.,0.,0.));
#38440=DIRECTION('center_axis',(0.,1.,0.));
#38441=DIRECTION('ref_axis',(0.,0.,-1.));
#38442=DIRECTION('',(0.,0.,-1.));
#38443=DIRECTION('',(-1.,0.,0.));
#38444=DIRECTION('',(0.,0.,-1.));
#38445=DIRECTION('center_axis',(0.,0.,1.));
#38446=DIRECTION('ref_axis',(0.,1.,0.));
#38447=DIRECTION('',(0.,1.,0.));
#38448=DIRECTION('',(-1.,0.,0.));
#38449=DIRECTION('',(0.,1.,0.));
#38450=DIRECTION('center_axis',(0.,-1.,0.));
#38451=DIRECTION('ref_axis',(0.,0.,1.));
#38452=DIRECTION('',(0.,0.,1.));
#38453=DIRECTION('',(0.,0.,1.));
#38454=DIRECTION('center_axis',(-1.,0.,0.));
#38455=DIRECTION('ref_axis',(0.,0.,1.));
#38456=DIRECTION('center_axis',(0.,0.,-1.));
#38457=DIRECTION('ref_axis',(0.,-1.,0.));
#38458=DIRECTION('',(0.,-1.,0.));
#38459=DIRECTION('',(-1.,0.,0.));
#38460=DIRECTION('',(0.,-1.,0.));
#38461=DIRECTION('',(-1.,0.,0.));
#38462=DIRECTION('center_axis',(0.,1.,0.));
#38463=DIRECTION('ref_axis',(0.,0.,-1.));
#38464=DIRECTION('',(0.,0.,-1.));
#38465=DIRECTION('',(-1.,0.,0.));
#38466=DIRECTION('',(0.,0.,-1.));
#38467=DIRECTION('center_axis',(0.,0.,1.));
#38468=DIRECTION('ref_axis',(0.,1.,0.));
#38469=DIRECTION('',(0.,1.,0.));
#38470=DIRECTION('',(-1.,0.,0.));
#38471=DIRECTION('',(0.,1.,0.));
#38472=DIRECTION('center_axis',(0.,-1.,0.));
#38473=DIRECTION('ref_axis',(0.,0.,1.));
#38474=DIRECTION('',(0.,0.,1.));
#38475=DIRECTION('',(0.,0.,1.));
#38476=DIRECTION('center_axis',(-1.,0.,0.));
#38477=DIRECTION('ref_axis',(0.,0.,1.));
#38478=DIRECTION('center_axis',(0.,0.,-1.));
#38479=DIRECTION('ref_axis',(0.,-1.,0.));
#38480=DIRECTION('',(0.,-1.,0.));
#38481=DIRECTION('',(-1.,0.,0.));
#38482=DIRECTION('',(0.,-1.,0.));
#38483=DIRECTION('',(-1.,0.,0.));
#38484=DIRECTION('center_axis',(0.,1.,0.));
#38485=DIRECTION('ref_axis',(0.,0.,-1.));
#38486=DIRECTION('',(0.,0.,-1.));
#38487=DIRECTION('',(-1.,0.,0.));
#38488=DIRECTION('',(0.,0.,-1.));
#38489=DIRECTION('center_axis',(0.,0.,1.));
#38490=DIRECTION('ref_axis',(0.,1.,0.));
#38491=DIRECTION('',(0.,1.,0.));
#38492=DIRECTION('',(-1.,0.,0.));
#38493=DIRECTION('',(0.,1.,0.));
#38494=DIRECTION('center_axis',(0.,-1.,0.));
#38495=DIRECTION('ref_axis',(0.,0.,1.));
#38496=DIRECTION('',(0.,0.,1.));
#38497=DIRECTION('',(0.,0.,1.));
#38498=DIRECTION('center_axis',(-1.,0.,0.));
#38499=DIRECTION('ref_axis',(0.,0.,1.));
#38500=DIRECTION('center_axis',(0.,0.,-1.));
#38501=DIRECTION('ref_axis',(0.,-1.,0.));
#38502=DIRECTION('',(0.,-1.,0.));
#38503=DIRECTION('',(-1.,0.,0.));
#38504=DIRECTION('',(0.,-1.,0.));
#38505=DIRECTION('',(-1.,0.,0.));
#38506=DIRECTION('center_axis',(0.,1.,0.));
#38507=DIRECTION('ref_axis',(0.,0.,-1.));
#38508=DIRECTION('',(0.,0.,-1.));
#38509=DIRECTION('',(-1.,0.,0.));
#38510=DIRECTION('',(0.,0.,-1.));
#38511=DIRECTION('center_axis',(0.,0.,1.));
#38512=DIRECTION('ref_axis',(0.,1.,0.));
#38513=DIRECTION('',(0.,1.,0.));
#38514=DIRECTION('',(-1.,0.,0.));
#38515=DIRECTION('',(0.,1.,0.));
#38516=DIRECTION('center_axis',(0.,-1.,0.));
#38517=DIRECTION('ref_axis',(0.,0.,1.));
#38518=DIRECTION('',(0.,0.,1.));
#38519=DIRECTION('',(0.,0.,1.));
#38520=DIRECTION('center_axis',(-1.,0.,0.));
#38521=DIRECTION('ref_axis',(0.,0.,1.));
#38522=DIRECTION('center_axis',(0.,0.,-1.));
#38523=DIRECTION('ref_axis',(0.,-1.,0.));
#38524=DIRECTION('',(0.,-1.,0.));
#38525=DIRECTION('',(-1.,0.,0.));
#38526=DIRECTION('',(0.,-1.,0.));
#38527=DIRECTION('',(-1.,0.,0.));
#38528=DIRECTION('center_axis',(0.,1.,0.));
#38529=DIRECTION('ref_axis',(0.,0.,-1.));
#38530=DIRECTION('',(0.,0.,-1.));
#38531=DIRECTION('',(-1.,0.,0.));
#38532=DIRECTION('',(0.,0.,-1.));
#38533=DIRECTION('center_axis',(0.,0.,1.));
#38534=DIRECTION('ref_axis',(0.,1.,0.));
#38535=DIRECTION('',(0.,1.,0.));
#38536=DIRECTION('',(-1.,0.,0.));
#38537=DIRECTION('',(0.,1.,0.));
#38538=DIRECTION('center_axis',(0.,-1.,0.));
#38539=DIRECTION('ref_axis',(0.,0.,1.));
#38540=DIRECTION('',(0.,0.,1.));
#38541=DIRECTION('',(0.,0.,1.));
#38542=DIRECTION('center_axis',(-1.,0.,0.));
#38543=DIRECTION('ref_axis',(0.,0.,1.));
#38544=DIRECTION('center_axis',(0.,0.,-1.));
#38545=DIRECTION('ref_axis',(0.,-1.,0.));
#38546=DIRECTION('',(0.,-1.,0.));
#38547=DIRECTION('',(-1.,0.,0.));
#38548=DIRECTION('',(0.,-1.,0.));
#38549=DIRECTION('',(-1.,0.,0.));
#38550=DIRECTION('center_axis',(0.,1.,0.));
#38551=DIRECTION('ref_axis',(0.,0.,-1.));
#38552=DIRECTION('',(0.,0.,-1.));
#38553=DIRECTION('',(-1.,0.,0.));
#38554=DIRECTION('',(0.,0.,-1.));
#38555=DIRECTION('center_axis',(0.,0.,1.));
#38556=DIRECTION('ref_axis',(0.,1.,0.));
#38557=DIRECTION('',(0.,1.,0.));
#38558=DIRECTION('',(-1.,0.,0.));
#38559=DIRECTION('',(0.,1.,0.));
#38560=DIRECTION('center_axis',(0.,-1.,0.));
#38561=DIRECTION('ref_axis',(0.,0.,1.));
#38562=DIRECTION('',(0.,0.,1.));
#38563=DIRECTION('',(0.,0.,1.));
#38564=DIRECTION('center_axis',(-1.,0.,0.));
#38565=DIRECTION('ref_axis',(0.,0.,1.));
#38566=DIRECTION('center_axis',(1.,0.,0.));
#38567=DIRECTION('ref_axis',(0.,0.,-1.));
#38568=DIRECTION('center_axis',(1.,0.,0.));
#38569=DIRECTION('ref_axis',(0.,0.,-1.));
#38570=DIRECTION('',(1.,0.,0.));
#38571=DIRECTION('center_axis',(-1.,0.,0.));
#38572=DIRECTION('ref_axis',(0.,0.,-1.));
#38573=DIRECTION('center_axis',(1.,0.,0.));
#38574=DIRECTION('ref_axis',(0.,0.,-1.));
#38575=DIRECTION('center_axis',(1.,0.,0.));
#38576=DIRECTION('ref_axis',(0.,0.,-1.));
#38577=DIRECTION('',(1.,0.,0.));
#38578=DIRECTION('center_axis',(-1.,0.,0.));
#38579=DIRECTION('ref_axis',(0.,0.,-1.));
#38580=DIRECTION('center_axis',(-1.,0.,0.));
#38581=DIRECTION('ref_axis',(0.,0.,1.));
#38582=DIRECTION('',(0.,0.,-1.));
#38583=DIRECTION('',(0.,1.,0.));
#38584=DIRECTION('',(0.,0.,1.));
#38585=DIRECTION('',(0.,1.,0.));
#38586=DIRECTION('center_axis',(0.,0.,-1.));
#38587=DIRECTION('ref_axis',(-1.,0.,0.));
#38588=DIRECTION('',(1.,0.,0.));
#38589=DIRECTION('',(-1.,0.,0.));
#38590=DIRECTION('',(0.,1.,0.));
#38591=DIRECTION('center_axis',(1.,0.,0.));
#38592=DIRECTION('ref_axis',(0.,0.,-1.));
#38593=DIRECTION('',(0.,0.,1.));
#38594=DIRECTION('',(0.,0.,-1.));
#38595=DIRECTION('',(0.,1.,0.));
#38596=DIRECTION('center_axis',(0.,0.,-1.));
#38597=DIRECTION('ref_axis',(-1.,0.,0.));
#38598=DIRECTION('',(1.,0.,0.));
#38599=DIRECTION('',(-1.,0.,0.));
#38600=DIRECTION('',(0.,1.,0.));
#38601=DIRECTION('center_axis',(-1.,0.,0.));
#38602=DIRECTION('ref_axis',(0.,0.,1.));
#38603=DIRECTION('',(0.,0.,-1.));
#38604=DIRECTION('',(0.,0.,1.));
#38605=DIRECTION('',(0.,1.,0.));
#38606=DIRECTION('center_axis',(0.,0.,-1.));
#38607=DIRECTION('ref_axis',(-1.,0.,0.));
#38608=DIRECTION('',(1.,0.,0.));
#38609=DIRECTION('',(-1.,0.,0.));
#38610=DIRECTION('',(0.,1.,0.));
#38611=DIRECTION('center_axis',(1.,0.,0.));
#38612=DIRECTION('ref_axis',(0.,0.,-1.));
#38613=DIRECTION('',(0.,0.,1.));
#38614=DIRECTION('',(0.,0.,-1.));
#38615=DIRECTION('',(0.,1.,0.));
#38616=DIRECTION('center_axis',(0.,0.,1.));
#38617=DIRECTION('ref_axis',(1.,0.,0.));
#38618=DIRECTION('',(-1.,0.,0.));
#38619=DIRECTION('',(1.,0.,0.));
#38620=DIRECTION('center_axis',(0.,1.,0.));
#38621=DIRECTION('ref_axis',(0.,0.,1.));
#38622=DIRECTION('center_axis',(0.,1.,0.));
#38623=DIRECTION('ref_axis',(1.,0.,0.));
#76648=CARTESIAN_POINT('',(0.,0.,0.));
#76649=CARTESIAN_POINT('Origin',(19.2,73.67,9.4));
#76650=CARTESIAN_POINT('',(19.2,73.67,9.4));
#76651=CARTESIAN_POINT('',(19.2,73.53,9.4));
#76652=CARTESIAN_POINT('',(19.2,68.835,9.4));
#76653=CARTESIAN_POINT('',(19.1,73.67,9.4));
#76654=CARTESIAN_POINT('',(19.2,73.67,9.4));
#76655=CARTESIAN_POINT('',(19.1,73.53,9.4));
#76656=CARTESIAN_POINT('',(19.1,73.53,9.4));
#76657=CARTESIAN_POINT('',(19.2,73.53,9.4));
#76658=CARTESIAN_POINT('Origin',(19.2,73.67,10.8));
#76659=CARTESIAN_POINT('',(19.2,73.67,10.8));
#76660=CARTESIAN_POINT('',(19.2,73.67,18.55));
#76661=CARTESIAN_POINT('',(19.1,73.67,10.8));
#76662=CARTESIAN_POINT('',(19.2,73.67,10.8));
#76663=CARTESIAN_POINT('',(19.1,73.67,9.4));
#76664=CARTESIAN_POINT('Origin',(19.2,73.53,10.8));
#76665=CARTESIAN_POINT('',(19.2,73.53,10.8));
#76666=CARTESIAN_POINT('',(19.2,68.765,10.8));
#76667=CARTESIAN_POINT('',(19.1,73.53,10.8));
#76668=CARTESIAN_POINT('',(19.2,73.53,10.8));
#76669=CARTESIAN_POINT('',(19.1,73.67,10.8));
#76670=CARTESIAN_POINT('Origin',(19.2,73.53,9.4));
#76671=CARTESIAN_POINT('',(19.2,73.53,17.85));
#76672=CARTESIAN_POINT('',(19.1,73.53,10.8));
#76673=CARTESIAN_POINT('Origin',(19.1,73.6,10.1));
#76674=CARTESIAN_POINT('Origin',(19.2,71.87,9.4));
#76675=CARTESIAN_POINT('',(19.2,71.87,9.4));
#76676=CARTESIAN_POINT('',(19.2,71.73,9.4));
#76677=CARTESIAN_POINT('',(19.2,67.935,9.4));
#76678=CARTESIAN_POINT('',(19.1,71.87,9.4));
#76679=CARTESIAN_POINT('',(19.2,71.87,9.4));
#76680=CARTESIAN_POINT('',(19.1,71.73,9.4));
#76681=CARTESIAN_POINT('',(19.1,71.73,9.4));
#76682=CARTESIAN_POINT('',(19.2,71.73,9.4));
#76683=CARTESIAN_POINT('Origin',(19.2,71.87,10.8));
#76684=CARTESIAN_POINT('',(19.2,71.87,10.8));
#76685=CARTESIAN_POINT('',(19.2,71.87,18.55));
#76686=CARTESIAN_POINT('',(19.1,71.87,10.8));
#76687=CARTESIAN_POINT('',(19.2,71.87,10.8));
#76688=CARTESIAN_POINT('',(19.1,71.87,9.4));
#76689=CARTESIAN_POINT('Origin',(19.2,71.73,10.8));
#76690=CARTESIAN_POINT('',(19.2,71.73,10.8));
#76691=CARTESIAN_POINT('',(19.2,67.865,10.8));
#76692=CARTESIAN_POINT('',(19.1,71.73,10.8));
#76693=CARTESIAN_POINT('',(19.2,71.73,10.8));
#76694=CARTESIAN_POINT('',(19.1,71.87,10.8));
#76695=CARTESIAN_POINT('Origin',(19.2,71.73,9.4));
#76696=CARTESIAN_POINT('',(19.2,71.73,17.85));
#76697=CARTESIAN_POINT('',(19.1,71.73,10.8));
#76698=CARTESIAN_POINT('Origin',(19.1,71.8,10.1));
#76699=CARTESIAN_POINT('Origin',(19.2,65.57,9.4));
#76700=CARTESIAN_POINT('',(19.2,65.57,9.4));
#76701=CARTESIAN_POINT('',(19.2,65.43,9.4));
#76702=CARTESIAN_POINT('',(19.2,64.785,9.4));
#76703=CARTESIAN_POINT('',(19.1,65.57,9.4));
#76704=CARTESIAN_POINT('',(19.2,65.57,9.4));
#76705=CARTESIAN_POINT('',(19.1,65.43,9.4));
#76706=CARTESIAN_POINT('',(19.1,65.43,9.4));
#76707=CARTESIAN_POINT('',(19.2,65.43,9.4));
#76708=CARTESIAN_POINT('Origin',(19.2,65.57,11.6));
#76709=CARTESIAN_POINT('',(19.2,65.57,11.6));
#76710=CARTESIAN_POINT('',(19.2,65.57,18.95));
#76711=CARTESIAN_POINT('',(19.1,65.57,11.6));
#76712=CARTESIAN_POINT('',(19.2,65.57,11.6));
#76713=CARTESIAN_POINT('',(19.1,65.57,9.4));
#76714=CARTESIAN_POINT('Origin',(19.2,65.43,11.6));
#76715=CARTESIAN_POINT('',(19.2,65.43,11.6));
#76716=CARTESIAN_POINT('',(19.2,64.715,11.6));
#76717=CARTESIAN_POINT('',(19.1,65.43,11.6));
#76718=CARTESIAN_POINT('',(19.2,65.43,11.6));
#76719=CARTESIAN_POINT('',(19.1,65.57,11.6));
#76720=CARTESIAN_POINT('Origin',(19.2,65.43,9.4));
#76721=CARTESIAN_POINT('',(19.2,65.43,17.85));
#76722=CARTESIAN_POINT('',(19.1,65.43,11.6));
#76723=CARTESIAN_POINT('Origin',(19.1,65.5,10.5));
#76724=CARTESIAN_POINT('Origin',(19.2,69.17,9.4));
#76725=CARTESIAN_POINT('',(19.2,69.17,9.4));
#76726=CARTESIAN_POINT('',(19.2,69.03,9.4));
#76727=CARTESIAN_POINT('',(19.2,66.585,9.4));
#76728=CARTESIAN_POINT('',(19.1,69.17,9.4));
#76729=CARTESIAN_POINT('',(19.2,69.17,9.4));
#76730=CARTESIAN_POINT('',(19.1,69.03,9.4));
#76731=CARTESIAN_POINT('',(19.1,69.03,9.4));
#76732=CARTESIAN_POINT('',(19.2,69.03,9.4));
#76733=CARTESIAN_POINT('Origin',(19.2,69.17,10.8));
#76734=CARTESIAN_POINT('',(19.2,69.17,10.8));
#76735=CARTESIAN_POINT('',(19.2,69.17,18.55));
#76736=CARTESIAN_POINT('',(19.1,69.17,10.8));
#76737=CARTESIAN_POINT('',(19.2,69.17,10.8));
#76738=CARTESIAN_POINT('',(19.1,69.17,9.4));
#76739=CARTESIAN_POINT('Origin',(19.2,69.03,10.8));
#76740=CARTESIAN_POINT('',(19.2,69.03,10.8));
#76741=CARTESIAN_POINT('',(19.2,66.515,10.8));
#76742=CARTESIAN_POINT('',(19.1,69.03,10.8));
#76743=CARTESIAN_POINT('',(19.2,69.03,10.8));
#76744=CARTESIAN_POINT('',(19.1,69.17,10.8));
#76745=CARTESIAN_POINT('Origin',(19.2,69.03,9.4));
#76746=CARTESIAN_POINT('',(19.2,69.03,17.85));
#76747=CARTESIAN_POINT('',(19.1,69.03,10.8));
#76748=CARTESIAN_POINT('Origin',(19.1,69.1,10.1));
#76749=CARTESIAN_POINT('Origin',(19.2,67.37,9.4));
#76750=CARTESIAN_POINT('',(19.2,67.37,9.4));
#76751=CARTESIAN_POINT('',(19.2,67.23,9.4));
#76752=CARTESIAN_POINT('',(19.2,65.685,9.4));
#76753=CARTESIAN_POINT('',(19.1,67.37,9.4));
#76754=CARTESIAN_POINT('',(19.2,67.37,9.4));
#76755=CARTESIAN_POINT('',(19.1,67.23,9.4));
#76756=CARTESIAN_POINT('',(19.1,67.23,9.4));
#76757=CARTESIAN_POINT('',(19.2,67.23,9.4));
#76758=CARTESIAN_POINT('Origin',(19.2,67.37,10.8));
#76759=CARTESIAN_POINT('',(19.2,67.37,10.8));
#76760=CARTESIAN_POINT('',(19.2,67.37,18.55));
#76761=CARTESIAN_POINT('',(19.1,67.37,10.8));
#76762=CARTESIAN_POINT('',(19.2,67.37,10.8));
#76763=CARTESIAN_POINT('',(19.1,67.37,9.4));
#76764=CARTESIAN_POINT('Origin',(19.2,67.23,10.8));
#76765=CARTESIAN_POINT('',(19.2,67.23,10.8));
#76766=CARTESIAN_POINT('',(19.2,65.615,10.8));
#76767=CARTESIAN_POINT('',(19.1,67.23,10.8));
#76768=CARTESIAN_POINT('',(19.2,67.23,10.8));
#76769=CARTESIAN_POINT('',(19.1,67.37,10.8));
#76770=CARTESIAN_POINT('Origin',(19.2,67.23,9.4));
#76771=CARTESIAN_POINT('',(19.2,67.23,17.85));
#76772=CARTESIAN_POINT('',(19.1,67.23,10.8));
#76773=CARTESIAN_POINT('Origin',(19.1,67.3,10.1));
#76774=CARTESIAN_POINT('Origin',(19.2,66.47,9.4));
#76775=CARTESIAN_POINT('',(19.2,66.47,9.4));
#76776=CARTESIAN_POINT('',(19.2,66.33,9.4));
#76777=CARTESIAN_POINT('',(19.2,65.235,9.4));
#76778=CARTESIAN_POINT('',(19.1,66.47,9.4));
#76779=CARTESIAN_POINT('',(19.2,66.47,9.4));
#76780=CARTESIAN_POINT('',(19.1,66.33,9.4));
#76781=CARTESIAN_POINT('',(19.1,66.33,9.4));
#76782=CARTESIAN_POINT('',(19.2,66.33,9.4));
#76783=CARTESIAN_POINT('Origin',(19.2,66.47,10.8));
#76784=CARTESIAN_POINT('',(19.2,66.47,10.8));
#76785=CARTESIAN_POINT('',(19.2,66.47,18.55));
#76786=CARTESIAN_POINT('',(19.1,66.47,10.8));
#76787=CARTESIAN_POINT('',(19.2,66.47,10.8));
#76788=CARTESIAN_POINT('',(19.1,66.47,9.4));
#76789=CARTESIAN_POINT('Origin',(19.2,66.33,10.8));
#76790=CARTESIAN_POINT('',(19.2,66.33,10.8));
#76791=CARTESIAN_POINT('',(19.2,65.165,10.8));
#76792=CARTESIAN_POINT('',(19.1,66.33,10.8));
#76793=CARTESIAN_POINT('',(19.2,66.33,10.8));
#76794=CARTESIAN_POINT('',(19.1,66.47,10.8));
#76795=CARTESIAN_POINT('Origin',(19.2,66.33,9.4));
#76796=CARTESIAN_POINT('',(19.2,66.33,17.85));
#76797=CARTESIAN_POINT('',(19.1,66.33,10.8));
#76798=CARTESIAN_POINT('Origin',(19.1,66.4,10.1));
#76799=CARTESIAN_POINT('Origin',(19.2,68.27,9.4));
#76800=CARTESIAN_POINT('',(19.2,68.27,9.4));
#76801=CARTESIAN_POINT('',(19.2,68.13,9.4));
#76802=CARTESIAN_POINT('',(19.2,66.135,9.4));
#76803=CARTESIAN_POINT('',(19.1,68.27,9.4));
#76804=CARTESIAN_POINT('',(19.2,68.27,9.4));
#76805=CARTESIAN_POINT('',(19.1,68.13,9.4));
#76806=CARTESIAN_POINT('',(19.1,68.13,9.4));
#76807=CARTESIAN_POINT('',(19.2,68.13,9.4));
#76808=CARTESIAN_POINT('Origin',(19.2,68.27,10.8));
#76809=CARTESIAN_POINT('',(19.2,68.27,10.8));
#76810=CARTESIAN_POINT('',(19.2,68.27,18.55));
#76811=CARTESIAN_POINT('',(19.1,68.27,10.8));
#76812=CARTESIAN_POINT('',(19.2,68.27,10.8));
#76813=CARTESIAN_POINT('',(19.1,68.27,9.4));
#76814=CARTESIAN_POINT('Origin',(19.2,68.13,10.8));
#76815=CARTESIAN_POINT('',(19.2,68.13,10.8));
#76816=CARTESIAN_POINT('',(19.2,66.065,10.8));
#76817=CARTESIAN_POINT('',(19.1,68.13,10.8));
#76818=CARTESIAN_POINT('',(19.2,68.13,10.8));
#76819=CARTESIAN_POINT('',(19.1,68.27,10.8));
#76820=CARTESIAN_POINT('Origin',(19.2,68.13,9.4));
#76821=CARTESIAN_POINT('',(19.2,68.13,17.85));
#76822=CARTESIAN_POINT('',(19.1,68.13,10.8));
#76823=CARTESIAN_POINT('Origin',(19.1,68.2,10.1));
#76824=CARTESIAN_POINT('Origin',(19.2,70.07,9.4));
#76825=CARTESIAN_POINT('',(19.2,70.07,9.4));
#76826=CARTESIAN_POINT('',(19.2,69.93,9.4));
#76827=CARTESIAN_POINT('',(19.2,67.035,9.4));
#76828=CARTESIAN_POINT('',(19.1,70.07,9.4));
#76829=CARTESIAN_POINT('',(19.2,70.07,9.4));
#76830=CARTESIAN_POINT('',(19.1,69.93,9.4));
#76831=CARTESIAN_POINT('',(19.1,69.93,9.4));
#76832=CARTESIAN_POINT('',(19.2,69.93,9.4));
#76833=CARTESIAN_POINT('Origin',(19.2,70.07,11.6));
#76834=CARTESIAN_POINT('',(19.2,70.07,11.6));
#76835=CARTESIAN_POINT('',(19.2,70.07,18.95));
#76836=CARTESIAN_POINT('',(19.1,70.07,11.6));
#76837=CARTESIAN_POINT('',(19.2,70.07,11.6));
#76838=CARTESIAN_POINT('',(19.1,70.07,9.4));
#76839=CARTESIAN_POINT('Origin',(19.2,69.93,11.6));
#76840=CARTESIAN_POINT('',(19.2,69.93,11.6));
#76841=CARTESIAN_POINT('',(19.2,66.965,11.6));
#76842=CARTESIAN_POINT('',(19.1,69.93,11.6));
#76843=CARTESIAN_POINT('',(19.2,69.93,11.6));
#76844=CARTESIAN_POINT('',(19.1,70.07,11.6));
#76845=CARTESIAN_POINT('Origin',(19.2,69.93,9.4));
#76846=CARTESIAN_POINT('',(19.2,69.93,17.85));
#76847=CARTESIAN_POINT('',(19.1,69.93,11.6));
#76848=CARTESIAN_POINT('Origin',(19.1,70.,10.5));
#76849=CARTESIAN_POINT('Origin',(19.2,70.97,9.4));
#76850=CARTESIAN_POINT('',(19.2,70.97,9.4));
#76851=CARTESIAN_POINT('',(19.2,70.83,9.4));
#76852=CARTESIAN_POINT('',(19.2,67.485,9.4));
#76853=CARTESIAN_POINT('',(19.1,70.97,9.4));
#76854=CARTESIAN_POINT('',(19.2,70.97,9.4));
#76855=CARTESIAN_POINT('',(19.1,70.83,9.4));
#76856=CARTESIAN_POINT('',(19.1,70.83,9.4));
#76857=CARTESIAN_POINT('',(19.2,70.83,9.4));
#76858=CARTESIAN_POINT('Origin',(19.2,70.97,10.8));
#76859=CARTESIAN_POINT('',(19.2,70.97,10.8));
#76860=CARTESIAN_POINT('',(19.2,70.97,18.55));
#76861=CARTESIAN_POINT('',(19.1,70.97,10.8));
#76862=CARTESIAN_POINT('',(19.2,70.97,10.8));
#76863=CARTESIAN_POINT('',(19.1,70.97,9.4));
#76864=CARTESIAN_POINT('Origin',(19.2,70.83,10.8));
#76865=CARTESIAN_POINT('',(19.2,70.83,10.8));
#76866=CARTESIAN_POINT('',(19.2,67.415,10.8));
#76867=CARTESIAN_POINT('',(19.1,70.83,10.8));
#76868=CARTESIAN_POINT('',(19.2,70.83,10.8));
#76869=CARTESIAN_POINT('',(19.1,70.97,10.8));
#76870=CARTESIAN_POINT('Origin',(19.2,70.83,9.4));
#76871=CARTESIAN_POINT('',(19.2,70.83,17.85));
#76872=CARTESIAN_POINT('',(19.1,70.83,10.8));
#76873=CARTESIAN_POINT('Origin',(19.1,70.9,10.1));
#76874=CARTESIAN_POINT('Origin',(19.2,72.77,9.4));
#76875=CARTESIAN_POINT('',(19.2,72.77,9.4));
#76876=CARTESIAN_POINT('',(19.2,72.63,9.4));
#76877=CARTESIAN_POINT('',(19.2,68.385,9.4));
#76878=CARTESIAN_POINT('',(19.1,72.77,9.4));
#76879=CARTESIAN_POINT('',(19.2,72.77,9.4));
#76880=CARTESIAN_POINT('',(19.1,72.63,9.4));
#76881=CARTESIAN_POINT('',(19.1,72.63,9.4));
#76882=CARTESIAN_POINT('',(19.2,72.63,9.4));
#76883=CARTESIAN_POINT('Origin',(19.2,72.77,10.8));
#76884=CARTESIAN_POINT('',(19.2,72.77,10.8));
#76885=CARTESIAN_POINT('',(19.2,72.77,18.55));
#76886=CARTESIAN_POINT('',(19.1,72.77,10.8));
#76887=CARTESIAN_POINT('',(19.2,72.77,10.8));
#76888=CARTESIAN_POINT('',(19.1,72.77,9.4));
#76889=CARTESIAN_POINT('Origin',(19.2,72.63,10.8));
#76890=CARTESIAN_POINT('',(19.2,72.63,10.8));
#76891=CARTESIAN_POINT('',(19.2,68.315,10.8));
#76892=CARTESIAN_POINT('',(19.1,72.63,10.8));
#76893=CARTESIAN_POINT('',(19.2,72.63,10.8));
#76894=CARTESIAN_POINT('',(19.1,72.77,10.8));
#76895=CARTESIAN_POINT('Origin',(19.2,72.63,9.4));
#76896=CARTESIAN_POINT('',(19.2,72.63,17.85));
#76897=CARTESIAN_POINT('',(19.1,72.63,10.8));
#76898=CARTESIAN_POINT('Origin',(19.1,72.7,10.1));
#76899=CARTESIAN_POINT('Origin',(19.2,74.57,9.4));
#76900=CARTESIAN_POINT('',(19.2,74.57,9.4));
#76901=CARTESIAN_POINT('',(19.2,74.43,9.4));
#76902=CARTESIAN_POINT('',(19.2,69.285,9.4));
#76903=CARTESIAN_POINT('',(19.1,74.57,9.4));
#76904=CARTESIAN_POINT('',(19.2,74.57,9.4));
#76905=CARTESIAN_POINT('',(19.1,74.43,9.4));
#76906=CARTESIAN_POINT('',(19.1,74.43,9.4));
#76907=CARTESIAN_POINT('',(19.2,74.43,9.4));
#76908=CARTESIAN_POINT('Origin',(19.2,74.57,11.6));
#76909=CARTESIAN_POINT('',(19.2,74.57,11.6));
#76910=CARTESIAN_POINT('',(19.2,74.57,18.95));
#76911=CARTESIAN_POINT('',(19.1,74.57,11.6));
#76912=CARTESIAN_POINT('',(19.2,74.57,11.6));
#76913=CARTESIAN_POINT('',(19.1,74.57,9.4));
#76914=CARTESIAN_POINT('Origin',(19.2,74.43,11.6));
#76915=CARTESIAN_POINT('',(19.2,74.43,11.6));
#76916=CARTESIAN_POINT('',(19.2,69.215,11.6));
#76917=CARTESIAN_POINT('',(19.1,74.43,11.6));
#76918=CARTESIAN_POINT('',(19.2,74.43,11.6));
#76919=CARTESIAN_POINT('',(19.1,74.57,11.6));
#76920=CARTESIAN_POINT('Origin',(19.2,74.43,9.4));
#76921=CARTESIAN_POINT('',(19.2,74.43,17.85));
#76922=CARTESIAN_POINT('',(19.1,74.43,11.6));
#76923=CARTESIAN_POINT('Origin',(19.1,74.5,10.5));
#76924=CARTESIAN_POINT('Origin',(12.5,67.,21.5));
#76925=CARTESIAN_POINT('',(12.5,67.,22.6));
#76926=CARTESIAN_POINT('Origin',(12.5,67.,21.5));
#76927=CARTESIAN_POINT('',(13.3,67.,22.6));
#76928=CARTESIAN_POINT('',(12.5,67.,22.6));
#76929=CARTESIAN_POINT('Origin',(13.3,67.,21.5));
#76930=CARTESIAN_POINT('Origin',(12.5,73.,21.5));
#76931=CARTESIAN_POINT('',(12.5,73.,22.6));
#76932=CARTESIAN_POINT('Origin',(12.5,73.,21.5));
#76933=CARTESIAN_POINT('',(13.3,73.,22.6));
#76934=CARTESIAN_POINT('',(12.5,73.,22.6));
#76935=CARTESIAN_POINT('Origin',(13.3,73.,21.5));
#76936=CARTESIAN_POINT('Origin',(12.5,64.,17.));
#76937=CARTESIAN_POINT('',(12.5,64.,26.3));
#76938=CARTESIAN_POINT('',(12.5,64.,17.));
#76939=CARTESIAN_POINT('',(12.5,64.,26.3));
#76940=CARTESIAN_POINT('',(12.5,76.,26.3));
#76941=CARTESIAN_POINT('',(12.5,64.,26.3));
#76942=CARTESIAN_POINT('',(12.5,76.,17.));
#76943=CARTESIAN_POINT('',(12.5,76.,26.3));
#76944=CARTESIAN_POINT('',(12.5,64.,17.));
#76945=CARTESIAN_POINT('Origin',(13.3,64.,17.));
#76946=CARTESIAN_POINT('',(13.3,64.,17.));
#76947=CARTESIAN_POINT('',(12.5,64.,17.));
#76948=CARTESIAN_POINT('',(13.3,76.,17.));
#76949=CARTESIAN_POINT('',(12.5,76.,17.));
#76950=CARTESIAN_POINT('',(13.3,64.,17.));
#76951=CARTESIAN_POINT('Origin',(13.3,64.,25.5));
#76952=CARTESIAN_POINT('',(13.3,64.,25.5));
#76953=CARTESIAN_POINT('',(13.3,64.,17.));
#76954=CARTESIAN_POINT('',(13.3,76.,25.5));
#76955=CARTESIAN_POINT('',(13.3,76.,17.));
#76956=CARTESIAN_POINT('',(13.3,64.,25.5));
#76957=CARTESIAN_POINT('Origin',(18.4,64.,25.5));
#76958=CARTESIAN_POINT('',(18.4,64.,25.5));
#76959=CARTESIAN_POINT('',(13.3,64.,25.5));
#76960=CARTESIAN_POINT('',(18.4,76.,25.5));
#76961=CARTESIAN_POINT('',(13.3,76.,25.5));
#76962=CARTESIAN_POINT('',(18.4,64.,25.5));
#76963=CARTESIAN_POINT('Origin',(18.4,64.,9.));
#76964=CARTESIAN_POINT('',(18.4,64.,9.));
#76965=CARTESIAN_POINT('',(18.4,64.,25.5));
#76966=CARTESIAN_POINT('',(18.4,76.,9.));
#76967=CARTESIAN_POINT('',(18.4,76.,25.5));
#76968=CARTESIAN_POINT('',(18.4,64.,9.));
#76969=CARTESIAN_POINT('Origin',(19.2,64.,9.));
#76970=CARTESIAN_POINT('',(19.2,64.,9.));
#76971=CARTESIAN_POINT('',(18.4,64.,9.));
#76972=CARTESIAN_POINT('',(19.2,76.,9.));
#76973=CARTESIAN_POINT('',(18.4,76.,9.));
#76974=CARTESIAN_POINT('',(19.2,64.,9.));
#76975=CARTESIAN_POINT('Origin',(19.2,64.,26.3));
#76976=CARTESIAN_POINT('',(19.2,64.,26.3));
#76977=CARTESIAN_POINT('',(19.2,64.,9.));
#76978=CARTESIAN_POINT('',(19.2,76.,26.3));
#76979=CARTESIAN_POINT('',(19.2,76.,9.));
#76980=CARTESIAN_POINT('',(19.2,64.,26.3));
#76981=CARTESIAN_POINT('Origin',(12.5,64.,26.3));
#76982=CARTESIAN_POINT('',(19.2,64.,26.3));
#76983=CARTESIAN_POINT('',(19.2,76.,26.3));
#76984=CARTESIAN_POINT('Origin',(15.85,76.,17.65));
#76985=CARTESIAN_POINT('Origin',(15.85,64.,17.65));
#135260=UNCERTAINTY_MEASURE_WITH_UNIT(LENGTH_MEASURE(0.01),#135283,
'DISTANCE_ACCURACY_VALUE',
'Maximum model space distance between geometric entities at asserted c
onnectivities');
#135267=UNCERTAINTY_MEASURE_WITH_UNIT(LENGTH_MEASURE(0.01),#135283,
'DISTANCE_ACCURACY_VALUE',
'Maximum model space distance between geometric entities at asserted c
onnectivities');
#135275=(
GEOMETRIC_REPRESENTATION_CONTEXT(3)
GLOBAL_UNCERTAINTY_ASSIGNED_CONTEXT((#135260))
GLOBAL_UNIT_ASSIGNED_CONTEXT((#135283,#135285,#135286))
REPRESENTATION_CONTEXT('','3D')
);
#135282=(
GEOMETRIC_REPRESENTATION_CONTEXT(3)
GLOBAL_UNCERTAINTY_ASSIGNED_CONTEXT((#135267))
GLOBAL_UNIT_ASSIGNED_CONTEXT((#135283,#135285,#135286))
REPRESENTATION_CONTEXT('','3D')
);
#135283=(
LENGTH_UNIT()
NAMED_UNIT(*)
SI_UNIT(.MILLI.,.METRE.)
);
#135285=(
NAMED_UNIT(*)
PLANE_ANGLE_UNIT()
SI_UNIT($,.RADIAN.)
);
#135286=(
NAMED_UNIT(*)
SI_UNIT($,.STERADIAN.)
SOLID_ANGLE_UNIT()
);
#135294=SHAPE_DEFINITION_REPRESENTATION(#135308,#135343);
#135308=PRODUCT_DEFINITION_SHAPE('',$,#135358);
#135343=SHAPE_REPRESENTATION('',(#33287),#135275);
#135350=PRODUCT_DEFINITION_CONTEXT('part definition',#135394,'design');
#135358=PRODUCT_DEFINITION('2026-10-15-19-09-11-262',
'Vernier Pointer Plate',#135372,#135350);
#135372=PRODUCT_DEFINITION_FORMATION('',$,#135403);
#135394=APPLICATION_CONTEXT(
'Core Data for Automotive Mechanical Design Process');
#135395=PRODUCT_CONTEXT('part definition',#135394,'mechanical');
#135403=PRODUCT('2026-10-15-19-09-11-262','Vernier Pointer Plate',$,(#135395));
#135417=PRESENTATION_STYLE_ASSIGNMENT((#135431));
#135431=SURFACE_STYLE_USAGE(.BOTH.,#135445);
#135445=SURFACE_SIDE_STYLE('',(#135459));
#135459=SURFACE_STYLE_FILL_AREA(#135473);
#135473=FILL_AREA_STYLE('Opaque(236,238,240)',(#135487));
#135487=FILL_AREA_STYLE_COLOUR('Opaque(236,238,240)',#135501);
#135501=COLOUR_RGB('Opaque(236,238,240)', 0.09019608, 0.27058824, 0.51372549);
ENDSEC;
END-ISO-10303-21;
